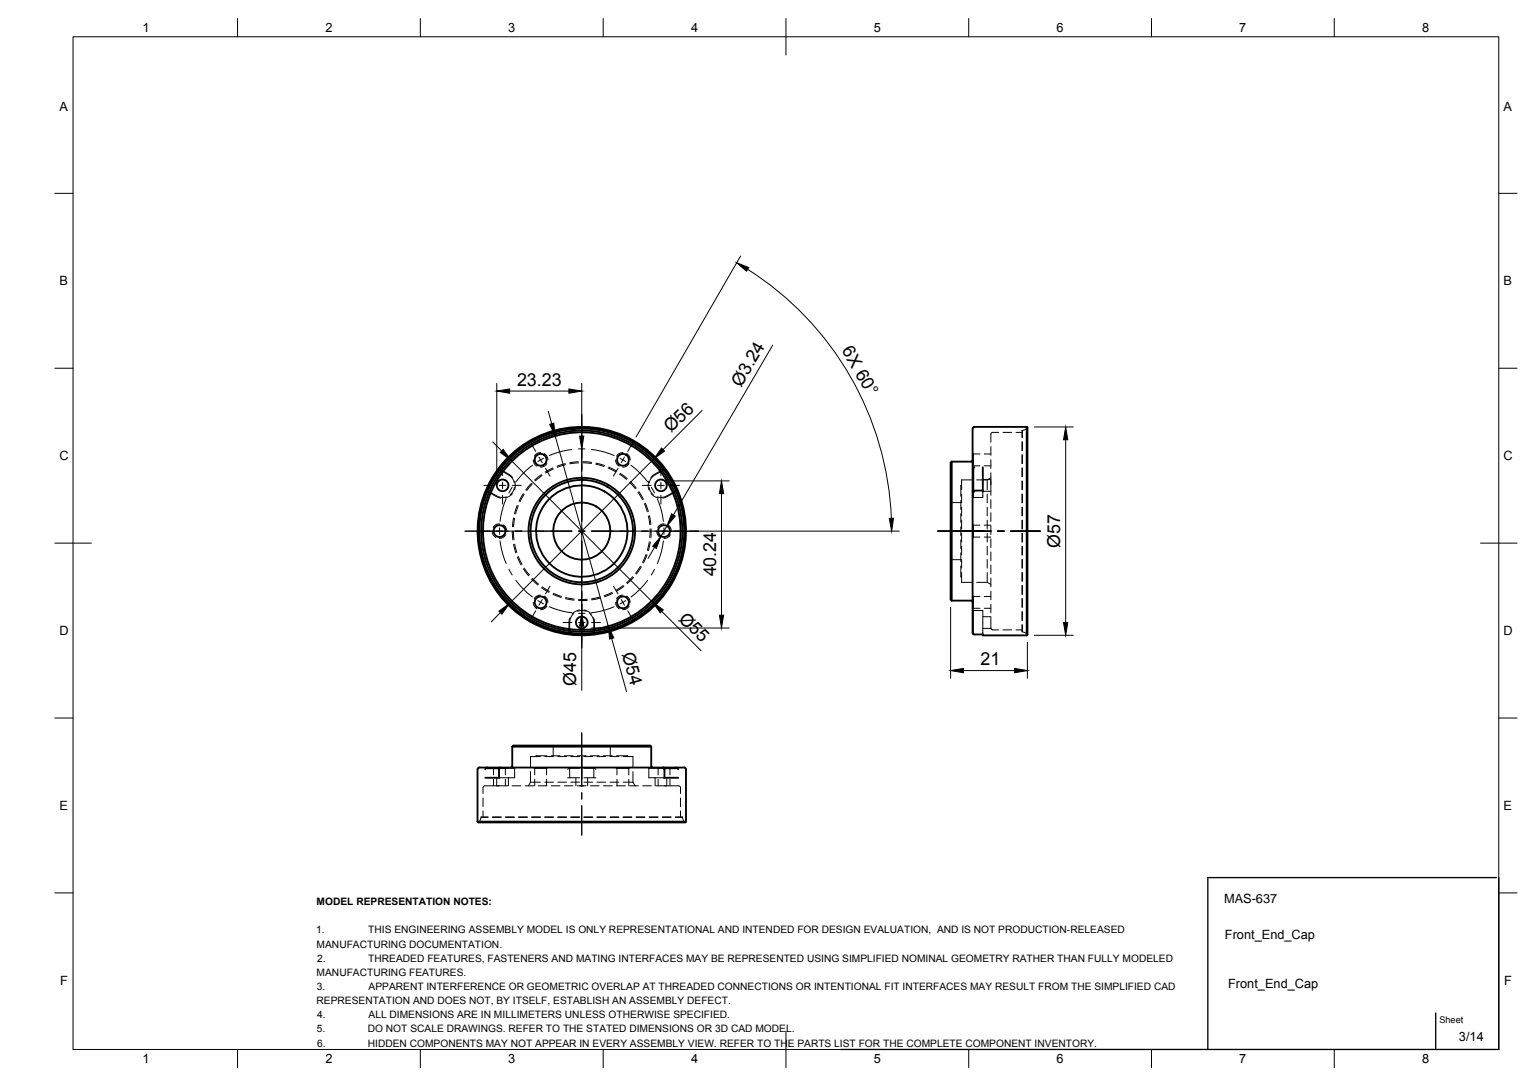
ISO-10303-21;
HEADER;
FILE_DESCRIPTION((''),'2;1');
FILE_NAME('Front_End_Cap.step','2026-10-09T10:11:57-07:00',(''),(''),'','','');
FILE_SCHEMA (('AUTOMOTIVE_DESIGN { 1 0 10303 214 3 1 1 }'));
ENDSEC;
DATA;
#10=MECHANICAL_DESIGN_GEOMETRIC_PRESENTATION_REPRESENTATION('',(#123),#13510);
#93=SHAPE_REPRESENTATION_RELATIONSHIP('SRR','None',#13563,#108) ;
#108=ADVANCED_BREP_SHAPE_REPRESENTATION('',(#155),#13495) ;
#123=STYLED_ITEM('',(#13647),#155) ;
#155=MANIFOLD_SOLID_BREP('Body1',#7372) ;
#187=ELLIPSE('',#7677,0.707106781186342,0.5) ;
#188=ELLIPSE('',#7688,0.707106781186342,0.5) ;
#189=ELLIPSE('',#7692,0.707106781186342,0.5) ;
#190=ELLIPSE('',#7702,0.707106781186342,0.5) ;
#191=ELLIPSE('',#7709,0.707106781186548,0.5) ;
#192=ELLIPSE('',#7716,0.707106781186548,0.5) ;
#193=FACE_BOUND('',#1127,.T.) ;
#194=FACE_BOUND('',#1131,.T.) ;
#195=FACE_BOUND('',#1137,.T.) ;
#196=FACE_BOUND('',#1140,.T.) ;
#197=FACE_BOUND('',#1143,.T.) ;
#198=FACE_BOUND('',#1150,.T.) ;
#199=FACE_BOUND('',#1151,.T.) ;
#200=FACE_BOUND('',#1152,.T.) ;
#201=FACE_BOUND('',#1153,.T.) ;
#202=FACE_BOUND('',#1154,.T.) ;
#203=FACE_BOUND('',#1155,.T.) ;
#204=FACE_BOUND('',#1156,.T.) ;
#205=FACE_BOUND('',#1173,.T.) ;
#206=FACE_BOUND('',#1174,.T.) ;
#207=FACE_BOUND('',#1175,.T.) ;
#208=FACE_BOUND('',#1176,.T.) ;
#209=FACE_BOUND('',#1177,.T.) ;
#210=FACE_BOUND('',#1178,.T.) ;
#211=FACE_BOUND('',#1179,.T.) ;
#212=FACE_BOUND('',#1185,.T.) ;
#213=FACE_BOUND('',#1194,.T.) ;
#214=FACE_BOUND('',#1204,.T.) ;
#266=PLANE('',#7586) ;
#267=PLANE('',#7592) ;
#268=PLANE('',#7604) ;
#269=PLANE('',#7608) ;
#270=PLANE('',#7612) ;
#271=PLANE('',#7630) ;
#272=PLANE('',#7669) ;
#273=PLANE('',#7675) ;
#274=PLANE('',#7676) ;
#275=PLANE('',#7680) ;
#276=PLANE('',#7686) ;
#277=PLANE('',#7687) ;
#278=PLANE('',#7690) ;
#279=PLANE('',#7691) ;
#280=PLANE('',#7695) ;
#281=PLANE('',#7700) ;
#282=PLANE('',#7701) ;
#283=PLANE('',#7707) ;
#284=PLANE('',#7708) ;
#285=PLANE('',#7712) ;
#286=PLANE('',#7714) ;
#287=PLANE('',#7715) ;
#474=B_SPLINE_CURVE_WITH_KNOTS('',3,(#11072,#11073,#11074,#11075,#11076,
#11077,#11078,#11079,#11080,#11081,#11082,#11083,#11084,#11085,#11086,#11087,
#11088,#11089,#11090,#11091,#11092,#11093),.UNSPECIFIED.,.F.,.F.,(4,2,2,
2,2,2,2,2,2,2,4),(-0.52146341780892,-0.494765818804412,-0.469284384601152,
-0.465421081717763,-0.463705360184221,-0.462435620950771,-0.461259293496834,
-0.45965735667046,-0.455678085608089,-0.412270185488608,-0.400473329912757),
 .UNSPECIFIED.) ;
#475=B_SPLINE_CURVE_WITH_KNOTS('',3,(#11097,#11098,#11099,#11100,#11101,
#11102,#11103,#11104,#11105,#11106,#11107,#11108,#11109,#11110,#11111,#11112,
#11113,#11114,#11115,#11116,#11117,#11118),.UNSPECIFIED.,.F.,.F.,(4,2,2,
2,2,2,2,2,2,2,4),(-0.521463417334395,-0.49476581835854,-0.469284384179659,
-0.465421081300331,-0.463705359768128,-0.462435620535193,-0.461259293081839,
-0.459657356256884,-0.455678085198087,-0.412270185114522,-0.400473329554445),
 .UNSPECIFIED.) ;
#476=B_SPLINE_CURVE_WITH_KNOTS('',3,(#11122,#11123,#11124,#11125,#11126,
#11127,#11128,#11129,#11130,#11131,#11132,#11133,#11134,#11135,#11136,#11137,
#11138,#11139,#11140,#11141,#11142,#11143),.UNSPECIFIED.,.F.,.F.,(4,2,2,
2,2,2,2,2,2,2,4),(-0.521463417713865,-0.494765818712896,-0.469284384508709,
-0.46542108162507,-0.463705360091333,-0.462435620857346,-0.461259293403164,
-0.459657356577429,-0.455678085515946,-0.412270185406787,-0.400473329829023),
 .UNSPECIFIED.) ;
#477=B_SPLINE_CURVE_WITH_KNOTS('',3,(#11350,#11351,#11352,#11353,#11354,
#11355),.UNSPECIFIED.,.F.,.F.,(4,2,4),(0.26873156819099,0.285572320159818,
0.298230301897838),.UNSPECIFIED.) ;
#478=B_SPLINE_CURVE_WITH_KNOTS('',3,(#11361,#11362,#11363,#11364,#11365,
#11366,#11367,#11368,#11369,#11370,#11371,#11372),.UNSPECIFIED.,.F.,.F.,
(4,2,2,2,2,4),(-0.000449132348290775,2.53732061403222E-12,0.0221149603912549,
0.0431990642467605,0.06500366116372,0.0651070090170544),.UNSPECIFIED.) ;
#479=B_SPLINE_CURVE_WITH_KNOTS('',3,(#11385,#11386,#11387,#11388,#11389,
#11390,#11391,#11392,#11393,#11394,#11395,#11396),.UNSPECIFIED.,.F.,.F.,
(4,2,2,2,2,4),(-0.000449133003127626,1.85615813084322E-12,0.0221149611703719,
0.0431990661916226,0.065003665298961,0.0651070140798856),.UNSPECIFIED.) ;
#480=B_SPLINE_CURVE_WITH_KNOTS('',3,(#11397,#11398,#11399,#11400,#11401,
#11402),.UNSPECIFIED.,.F.,.F.,(4,2,4),(-0.0927109544955969,-0.0758702025273432,
-0.0632122207848772),.UNSPECIFIED.) ;
#481=B_SPLINE_CURVE_WITH_KNOTS('',3,(#11404,#11405,#11406,#11407,#11408,
#11409),.UNSPECIFIED.,.F.,.F.,(4,2,4),(0.268765463242126,0.285606215210891,
0.298264196947108),.UNSPECIFIED.) ;
#482=B_SPLINE_CURVE_WITH_KNOTS('',3,(#11411,#11412,#11413,#11414,#11415,
#11416,#11417,#11418,#11419,#11420,#11421,#11422),.UNSPECIFIED.,.F.,.F.,
(4,2,2,2,2,4),(-0.22538340226828,-0.224833171566157,-0.19774023813781,-0.171910201657709,
-0.145197491309789,-0.145070879202733),.UNSPECIFIED.) ;
#483=B_SPLINE_CURVE_WITH_KNOTS('',3,(#11455,#11456,#11457,#11458,#11459,
#11460,#11461,#11462,#11463,#11464,#11465,#11466),.UNSPECIFIED.,.F.,.F.,
(4,2,2,2,2,4),(-0.000449132829525576,1.42051192857096E-13,0.0221149610887194,
0.0431990659374438,0.0650036645796739,0.0651070130619044),.UNSPECIFIED.) ;
#484=B_SPLINE_CURVE_WITH_KNOTS('',3,(#11467,#11468,#11469,#11470,#11471,
#11472),.UNSPECIFIED.,.F.,.F.,(4,2,4),(-0.0927109544901547,-0.0758702025249889,
-0.0632122207639069),.UNSPECIFIED.) ;
#485=B_SPLINE_CURVE_WITH_KNOTS('',3,(#11474,#11475,#11476,#11477,#11478,
#11479),.UNSPECIFIED.,.F.,.F.,(4,2,4),(0.268731568191897,0.285572320160214,
0.298230301904486),.UNSPECIFIED.) ;
#486=B_SPLINE_CURVE_WITH_KNOTS('',3,(#11480,#11481,#11482,#11483,#11484,
#11485,#11486,#11487,#11488,#11489,#11490,#11491),.UNSPECIFIED.,.F.,.F.,
(4,2,2,2,2,4),(-0.225383330725163,-0.224833100967517,-0.197740175527576,
-0.171910147180953,-0.145197446451029,-0.145070835530411),.UNSPECIFIED.) ;
#487=B_SPLINE_CURVE_WITH_KNOTS('',3,(#11529,#11530,#11531,#11532,#11533,
#11534),.UNSPECIFIED.,.F.,.F.,(4,2,4),(-0.0927254732348807,-0.0743662922611468,
-0.0631177306127901),.UNSPECIFIED.) ;
#488=B_SPLINE_CURVE_WITH_KNOTS('',3,(#11537,#11538,#11539,#11540,#11541,
#11542,#11543,#11544,#11545,#11546,#11547,#11548),.UNSPECIFIED.,.F.,.F.,
(4,2,2,2,2,4),(-0.225383401816229,-0.224833171320864,-0.197740237586304,
-0.171910200932329,-0.145197490755643,-0.145070879020991),.UNSPECIFIED.) ;
#492=TOROIDAL_SURFACE('',#7577,26.5,0.5) ;
#493=TOROIDAL_SURFACE('',#7596,19.4,0.4) ;
#494=TOROIDAL_SURFACE('',#7683,28.,0.5) ;
#495=TOROIDAL_SURFACE('',#7698,28.,0.5) ;
#496=TOROIDAL_SURFACE('',#7717,28.,0.5) ;
#541=CYLINDRICAL_SURFACE('',#7575,1.621) ;
#542=CYLINDRICAL_SURFACE('',#7584,27.) ;
#543=CYLINDRICAL_SURFACE('',#7588,27.5) ;
#544=CYLINDRICAL_SURFACE('',#7600,19.) ;
#545=CYLINDRICAL_SURFACE('',#7606,7.8) ;
#546=CYLINDRICAL_SURFACE('',#7610,12.5) ;
#547=CYLINDRICAL_SURFACE('',#7614,14.) ;
#548=CYLINDRICAL_SURFACE('',#7618,1.6) ;
#549=CYLINDRICAL_SURFACE('',#7622,1.6) ;
#550=CYLINDRICAL_SURFACE('',#7626,1.6) ;
#551=CYLINDRICAL_SURFACE('',#7639,1.621) ;
#552=CYLINDRICAL_SURFACE('',#7643,1.621) ;
#553=CYLINDRICAL_SURFACE('',#7647,1.621) ;
#554=CYLINDRICAL_SURFACE('',#7651,1.621) ;
#555=CYLINDRICAL_SURFACE('',#7655,1.621) ;
#556=CYLINDRICAL_SURFACE('',#7656,3.3) ;
#557=CYLINDRICAL_SURFACE('',#7661,3.3) ;
#558=CYLINDRICAL_SURFACE('',#7666,3.3) ;
#559=CYLINDRICAL_SURFACE('',#7678,0.5) ;
#560=CYLINDRICAL_SURFACE('',#7689,0.5) ;
#561=CYLINDRICAL_SURFACE('',#7693,0.5) ;
#562=CYLINDRICAL_SURFACE('',#7703,28.5) ;
#563=CYLINDRICAL_SURFACE('',#7706,0.5) ;
#564=CYLINDRICAL_SURFACE('',#7710,0.5) ;
#565=CYLINDRICAL_SURFACE('',#7718,0.5) ;
#668=FACE_OUTER_BOUND('',#1122,.T.) ;
#669=FACE_OUTER_BOUND('',#1123,.T.) ;
#670=FACE_OUTER_BOUND('',#1124,.T.) ;
#671=FACE_OUTER_BOUND('',#1125,.T.) ;
#672=FACE_OUTER_BOUND('',#1126,.T.) ;
#673=FACE_OUTER_BOUND('',#1128,.T.) ;
#674=FACE_OUTER_BOUND('',#1129,.T.) ;
#675=FACE_OUTER_BOUND('',#1130,.T.) ;
#676=FACE_OUTER_BOUND('',#1132,.T.) ;
#677=FACE_OUTER_BOUND('',#1133,.T.) ;
#678=FACE_OUTER_BOUND('',#1134,.T.) ;
#679=FACE_OUTER_BOUND('',#1135,.T.) ;
#680=FACE_OUTER_BOUND('',#1136,.T.) ;
#681=FACE_OUTER_BOUND('',#1138,.T.) ;
#682=FACE_OUTER_BOUND('',#1139,.T.) ;
#683=FACE_OUTER_BOUND('',#1141,.T.) ;
#684=FACE_OUTER_BOUND('',#1142,.T.) ;
#685=FACE_OUTER_BOUND('',#1144,.T.) ;
#686=FACE_OUTER_BOUND('',#1145,.T.) ;
#687=FACE_OUTER_BOUND('',#1146,.T.) ;
#688=FACE_OUTER_BOUND('',#1147,.T.) ;
#689=FACE_OUTER_BOUND('',#1148,.T.) ;
#690=FACE_OUTER_BOUND('',#1149,.T.) ;
#691=FACE_OUTER_BOUND('',#1157,.T.) ;
#692=FACE_OUTER_BOUND('',#1158,.T.) ;
#693=FACE_OUTER_BOUND('',#1159,.T.) ;
#694=FACE_OUTER_BOUND('',#1160,.T.) ;
#695=FACE_OUTER_BOUND('',#1161,.T.) ;
#696=FACE_OUTER_BOUND('',#1162,.T.) ;
#697=FACE_OUTER_BOUND('',#1163,.T.) ;
#698=FACE_OUTER_BOUND('',#1164,.T.) ;
#699=FACE_OUTER_BOUND('',#1165,.T.) ;
#700=FACE_OUTER_BOUND('',#1166,.T.) ;
#701=FACE_OUTER_BOUND('',#1167,.T.) ;
#702=FACE_OUTER_BOUND('',#1168,.T.) ;
#703=FACE_OUTER_BOUND('',#1169,.T.) ;
#704=FACE_OUTER_BOUND('',#1170,.T.) ;
#705=FACE_OUTER_BOUND('',#1171,.T.) ;
#706=FACE_OUTER_BOUND('',#1172,.T.) ;
#707=FACE_OUTER_BOUND('',#1180,.T.) ;
#708=FACE_OUTER_BOUND('',#1181,.T.) ;
#709=FACE_OUTER_BOUND('',#1182,.T.) ;
#710=FACE_OUTER_BOUND('',#1183,.T.) ;
#711=FACE_OUTER_BOUND('',#1184,.T.) ;
#712=FACE_OUTER_BOUND('',#1186,.T.) ;
#713=FACE_OUTER_BOUND('',#1187,.T.) ;
#714=FACE_OUTER_BOUND('',#1188,.T.) ;
#715=FACE_OUTER_BOUND('',#1189,.T.) ;
#716=FACE_OUTER_BOUND('',#1190,.T.) ;
#717=FACE_OUTER_BOUND('',#1191,.T.) ;
#718=FACE_OUTER_BOUND('',#1192,.T.) ;
#719=FACE_OUTER_BOUND('',#1193,.T.) ;
#720=FACE_OUTER_BOUND('',#1195,.T.) ;
#721=FACE_OUTER_BOUND('',#1196,.T.) ;
#722=FACE_OUTER_BOUND('',#1197,.T.) ;
#723=FACE_OUTER_BOUND('',#1198,.T.) ;
#724=FACE_OUTER_BOUND('',#1199,.T.) ;
#725=FACE_OUTER_BOUND('',#1200,.T.) ;
#726=FACE_OUTER_BOUND('',#1201,.T.) ;
#727=FACE_OUTER_BOUND('',#1202,.T.) ;
#728=FACE_OUTER_BOUND('',#1203,.T.) ;
#729=FACE_OUTER_BOUND('',#1205,.T.) ;
#730=FACE_OUTER_BOUND('',#1206,.T.) ;
#731=FACE_OUTER_BOUND('',#1207,.T.) ;
#732=FACE_OUTER_BOUND('',#1208,.T.) ;
#1122=EDGE_LOOP('',(#4822,#4823,#4824,#4825)) ;
#1123=EDGE_LOOP('',(#4826,#4827,#4828,#4829)) ;
#1124=EDGE_LOOP('',(#4830,#4831,#4832,#4833,#4834,#4835,#4836,#4837,#4838,
#4839)) ;
#1125=EDGE_LOOP('',(#4840,#4841,#4842,#4843)) ;
#1126=EDGE_LOOP('',(#4844)) ;
#1127=EDGE_LOOP('',(#4845)) ;
#1128=EDGE_LOOP('',(#4846,#4847,#4848,#4849)) ;
#1129=EDGE_LOOP('',(#4850,#4851,#4852,#4853)) ;
#1130=EDGE_LOOP('',(#4854)) ;
#1131=EDGE_LOOP('',(#4855)) ;
#1132=EDGE_LOOP('',(#4856,#4857,#4858,#4859)) ;
#1133=EDGE_LOOP('',(#4860,#4861,#4862,#4863)) ;
#1134=EDGE_LOOP('',(#4864,#4865,#4866,#4867)) ;
#1135=EDGE_LOOP('',(#4868,#4869,#4870,#4871)) ;
#1136=EDGE_LOOP('',(#4872)) ;
#1137=EDGE_LOOP('',(#4873)) ;
#1138=EDGE_LOOP('',(#4874,#4875,#4876,#4877)) ;
#1139=EDGE_LOOP('',(#4878)) ;
#1140=EDGE_LOOP('',(#4879)) ;
#1141=EDGE_LOOP('',(#4880,#4881,#4882,#4883)) ;
#1142=EDGE_LOOP('',(#4884)) ;
#1143=EDGE_LOOP('',(#4885)) ;
#1144=EDGE_LOOP('',(#4886,#4887,#4888,#4889)) ;
#1145=EDGE_LOOP('',(#4890,#4891,#4892,#4893)) ;
#1146=EDGE_LOOP('',(#4894,#4895,#4896,#4897,#4898,#4899)) ;
#1147=EDGE_LOOP('',(#4900,#4901,#4902,#4903,#4904,#4905)) ;
#1148=EDGE_LOOP('',(#4906,#4907,#4908,#4909,#4910,#4911)) ;
#1149=EDGE_LOOP('',(#4912,#4913,#4914,#4915,#4916,#4917,#4918,#4919,#4920,
#4921)) ;
#1150=EDGE_LOOP('',(#4922)) ;
#1151=EDGE_LOOP('',(#4923)) ;
#1152=EDGE_LOOP('',(#4924)) ;
#1153=EDGE_LOOP('',(#4925)) ;
#1154=EDGE_LOOP('',(#4926)) ;
#1155=EDGE_LOOP('',(#4927)) ;
#1156=EDGE_LOOP('',(#4928)) ;
#1157=EDGE_LOOP('',(#4929,#4930,#4931,#4932)) ;
#1158=EDGE_LOOP('',(#4933,#4934,#4935,#4936)) ;
#1159=EDGE_LOOP('',(#4937,#4938,#4939,#4940)) ;
#1160=EDGE_LOOP('',(#4941,#4942,#4943,#4944)) ;
#1161=EDGE_LOOP('',(#4945,#4946,#4947,#4948)) ;
#1162=EDGE_LOOP('',(#4949,#4950,#4951,#4952)) ;
#1163=EDGE_LOOP('',(#4953,#4954,#4955,#4956)) ;
#1164=EDGE_LOOP('',(#4957,#4958,#4959,#4960)) ;
#1165=EDGE_LOOP('',(#4961,#4962,#4963,#4964)) ;
#1166=EDGE_LOOP('',(#4965,#4966,#4967,#4968)) ;
#1167=EDGE_LOOP('',(#4969,#4970,#4971,#4972)) ;
#1168=EDGE_LOOP('',(#4973,#4974,#4975,#4976)) ;
#1169=EDGE_LOOP('',(#4977,#4978,#4979,#4980)) ;
#1170=EDGE_LOOP('',(#4981,#4982,#4983,#4984)) ;
#1171=EDGE_LOOP('',(#4985,#4986,#4987,#4988)) ;
#1172=EDGE_LOOP('',(#4989,#4990,#4991,#4992,#4993,#4994,#4995,#4996,#4997,
#4998,#4999,#5000)) ;
#1173=EDGE_LOOP('',(#5001)) ;
#1174=EDGE_LOOP('',(#5002)) ;
#1175=EDGE_LOOP('',(#5003)) ;
#1176=EDGE_LOOP('',(#5004)) ;
#1177=EDGE_LOOP('',(#5005)) ;
#1178=EDGE_LOOP('',(#5006)) ;
#1179=EDGE_LOOP('',(#5007)) ;
#1180=EDGE_LOOP('',(#5008,#5009,#5010,#5011)) ;
#1181=EDGE_LOOP('',(#5012,#5013,#5014,#5015)) ;
#1182=EDGE_LOOP('',(#5016,#5017,#5018,#5019,#5020)) ;
#1183=EDGE_LOOP('',(#5021,#5022,#5023,#5024,#5025)) ;
#1184=EDGE_LOOP('',(#5026,#5027,#5028,#5029,#5030,#5031)) ;
#1185=EDGE_LOOP('',(#5032)) ;
#1186=EDGE_LOOP('',(#5033,#5034,#5035,#5036,#5037,#5038,#5039)) ;
#1187=EDGE_LOOP('',(#5040,#5041,#5042,#5043)) ;
#1188=EDGE_LOOP('',(#5044,#5045,#5046,#5047,#5048)) ;
#1189=EDGE_LOOP('',(#5049,#5050,#5051,#5052,#5053)) ;
#1190=EDGE_LOOP('',(#5054,#5055,#5056,#5057)) ;
#1191=EDGE_LOOP('',(#5058,#5059,#5060,#5061,#5062)) ;
#1192=EDGE_LOOP('',(#5063,#5064,#5065,#5066,#5067)) ;
#1193=EDGE_LOOP('',(#5068,#5069,#5070,#5071,#5072,#5073)) ;
#1194=EDGE_LOOP('',(#5074)) ;
#1195=EDGE_LOOP('',(#5075,#5076,#5077,#5078,#5079,#5080)) ;
#1196=EDGE_LOOP('',(#5081,#5082,#5083,#5084)) ;
#1197=EDGE_LOOP('',(#5085,#5086,#5087,#5088,#5089)) ;
#1198=EDGE_LOOP('',(#5090,#5091,#5092,#5093,#5094,#5095,#5096,#5097,#5098,
#5099,#5100,#5101,#5102,#5103,#5104,#5105)) ;
#1199=EDGE_LOOP('',(#5106,#5107,#5108,#5109,#5110)) ;
#1200=EDGE_LOOP('',(#5111,#5112,#5113,#5114)) ;
#1201=EDGE_LOOP('',(#5115,#5116,#5117,#5118,#5119)) ;
#1202=EDGE_LOOP('',(#5120,#5121,#5122,#5123,#5124)) ;
#1203=EDGE_LOOP('',(#5125,#5126,#5127,#5128,#5129,#5130)) ;
#1204=EDGE_LOOP('',(#5131)) ;
#1205=EDGE_LOOP('',(#5132,#5133,#5134,#5135)) ;
#1206=EDGE_LOOP('',(#5136,#5137,#5138,#5139,#5140)) ;
#1207=EDGE_LOOP('',(#5141,#5142,#5143,#5144,#5145,#5146)) ;
#1208=EDGE_LOOP('',(#5147,#5148,#5149,#5150,#5151)) ;
#1649=LINE('',#11061,#2143) ;
#1650=LINE('',#11065,#2144) ;
#1651=LINE('',#11150,#2145) ;
#1652=LINE('',#11157,#2146) ;
#1653=LINE('',#11161,#2147) ;
#1654=LINE('',#11169,#2148) ;
#1655=LINE('',#11178,#2149) ;
#1656=LINE('',#11182,#2150) ;
#1657=LINE('',#11189,#2151) ;
#1658=LINE('',#11196,#2152) ;
#1659=LINE('',#11203,#2153) ;
#1660=LINE('',#11207,#2154) ;
#1661=LINE('',#11213,#2155) ;
#1662=LINE('',#11220,#2156) ;
#1663=LINE('',#11227,#2157) ;
#1664=LINE('',#11245,#2158) ;
#1665=LINE('',#11248,#2159) ;
#1666=LINE('',#11253,#2160) ;
#1667=LINE('',#11256,#2161) ;
#1668=LINE('',#11261,#2162) ;
#1669=LINE('',#11264,#2163) ;
#1670=LINE('',#11269,#2164) ;
#1671=LINE('',#11272,#2165) ;
#1672=LINE('',#11277,#2166) ;
#1673=LINE('',#11280,#2167) ;
#1674=LINE('',#11286,#2168) ;
#1675=LINE('',#11289,#2169) ;
#1676=LINE('',#11292,#2170) ;
#1677=LINE('',#11294,#2171) ;
#1678=LINE('',#11301,#2172) ;
#1679=LINE('',#11304,#2173) ;
#1680=LINE('',#11307,#2174) ;
#1681=LINE('',#11309,#2175) ;
#1682=LINE('',#11316,#2176) ;
#1683=LINE('',#11319,#2177) ;
#1684=LINE('',#11323,#2178) ;
#1685=LINE('',#11327,#2179) ;
#1686=LINE('',#11330,#2180) ;
#1687=LINE('',#11332,#2181) ;
#1688=LINE('',#11335,#2182) ;
#1689=LINE('',#11337,#2183) ;
#1690=LINE('',#11340,#2184) ;
#1691=LINE('',#11341,#2185) ;
#1692=LINE('',#11344,#2186) ;
#1693=LINE('',#11346,#2187) ;
#1694=LINE('',#11347,#2188) ;
#1695=LINE('',#11373,#2189) ;
#1696=LINE('',#11376,#2190) ;
#1697=LINE('',#11426,#2191) ;
#1698=LINE('',#11427,#2192) ;
#1699=LINE('',#11431,#2193) ;
#1700=LINE('',#11434,#2194) ;
#1701=LINE('',#11436,#2195) ;
#1702=LINE('',#11437,#2196) ;
#1703=LINE('',#11443,#2197) ;
#1704=LINE('',#11446,#2198) ;
#1705=LINE('',#11494,#2199) ;
#1706=LINE('',#11495,#2200) ;
#1707=LINE('',#11499,#2201) ;
#1708=LINE('',#11503,#2202) ;
#1709=LINE('',#11506,#2203) ;
#1710=LINE('',#11507,#2204) ;
#1711=LINE('',#11511,#2205) ;
#1712=LINE('',#11513,#2206) ;
#1713=LINE('',#11514,#2207) ;
#1714=LINE('',#11521,#2208) ;
#1715=LINE('',#11525,#2209) ;
#1716=LINE('',#11526,#2210) ;
#2143=VECTOR('',#8575,1.621) ;
#2144=VECTOR('',#8580,1.621) ;
#2145=VECTOR('',#8599,27.) ;
#2146=VECTOR('',#8608,27.5) ;
#2147=VECTOR('',#8613,27.5) ;
#2148=VECTOR('',#8624,28.3) ;
#2149=VECTOR('',#8635,19.) ;
#2150=VECTOR('',#8640,18.7) ;
#2151=VECTOR('',#8649,7.8) ;
#2152=VECTOR('',#8658,12.5) ;
#2153=VECTOR('',#8667,14.) ;
#2154=VECTOR('',#8672,14.) ;
#2155=VECTOR('',#8679,1.6) ;
#2156=VECTOR('',#8688,1.6) ;
#2157=VECTOR('',#8697,1.6) ;
#2158=VECTOR('',#8718,1.621) ;
#2159=VECTOR('',#8723,1.621) ;
#2160=VECTOR('',#8728,1.621) ;
#2161=VECTOR('',#8733,1.621) ;
#2162=VECTOR('',#8738,1.621) ;
#2163=VECTOR('',#8743,1.621) ;
#2164=VECTOR('',#8748,1.621) ;
#2165=VECTOR('',#8753,1.621) ;
#2166=VECTOR('',#8758,1.621) ;
#2167=VECTOR('',#8763,1.621) ;
#2168=VECTOR('',#8768,1.) ;
#2169=VECTOR('',#8771,1.) ;
#2170=VECTOR('',#8774,0.999999999999642) ;
#2171=VECTOR('',#8775,1.00000000000035) ;
#2172=VECTOR('',#8782,1.) ;
#2173=VECTOR('',#8785,1.) ;
#2174=VECTOR('',#8788,0.999999999999642) ;
#2175=VECTOR('',#8789,0.999999999999901) ;
#2176=VECTOR('',#8796,1.) ;
#2177=VECTOR('',#8799,1.) ;
#2178=VECTOR('',#8802,1.) ;
#2179=VECTOR('',#8805,1.) ;
#2180=VECTOR('',#8808,0.99999999999962) ;
#2181=VECTOR('',#8809,0.99999999999962) ;
#2182=VECTOR('',#8812,0.99999999999962) ;
#2183=VECTOR('',#8813,0.99999999999962) ;
#2184=VECTOR('',#8818,0.999999999999933) ;
#2185=VECTOR('',#8819,0.999999999999933) ;
#2186=VECTOR('',#8822,0.99999999999962) ;
#2187=VECTOR('',#8823,0.99999999999962) ;
#2188=VECTOR('',#8824,1.) ;
#2189=VECTOR('',#8833,1.) ;
#2190=VECTOR('',#8836,0.99999999999962) ;
#2191=VECTOR('',#8849,0.99999999999962) ;
#2192=VECTOR('',#8850,1.) ;
#2193=VECTOR('',#8857,1.) ;
#2194=VECTOR('',#8860,0.99999999999962) ;
#2195=VECTOR('',#8861,0.99999999999962) ;
#2196=VECTOR('',#8862,1.) ;
#2197=VECTOR('',#8871,1.) ;
#2198=VECTOR('',#8874,0.99999999999962) ;
#2199=VECTOR('',#8885,0.99999999999962) ;
#2200=VECTOR('',#8886,1.) ;
#2201=VECTOR('',#8893,28.5) ;
#2202=VECTOR('',#8896,1.) ;
#2203=VECTOR('',#8899,1.) ;
#2204=VECTOR('',#8900,1.) ;
#2205=VECTOR('',#8905,1.) ;
#2206=VECTOR('',#8906,1.) ;
#2207=VECTOR('',#8907,1.) ;
#2208=VECTOR('',#8918,1.) ;
#2209=VECTOR('',#8923,1.) ;
#2210=VECTOR('',#8924,1.) ;
#2637=CIRCLE('',#7573,1.621) ;
#2638=CIRCLE('',#7574,2.) ;
#2639=CIRCLE('',#7576,1.621) ;
#2640=CIRCLE('',#7578,26.5) ;
#2641=CIRCLE('',#7579,26.5) ;
#2642=CIRCLE('',#7580,26.5) ;
#2643=CIRCLE('',#7581,26.5) ;
#2644=CIRCLE('',#7582,0.5) ;
#2645=CIRCLE('',#7583,27.) ;
#2646=CIRCLE('',#7585,27.) ;
#2647=CIRCLE('',#7587,27.5) ;
#2648=CIRCLE('',#7589,27.5) ;
#2649=CIRCLE('',#7591,28.) ;
#2650=CIRCLE('',#7593,28.3) ;
#2651=CIRCLE('',#7595,28.5) ;
#2652=CIRCLE('',#7597,19.4) ;
#2653=CIRCLE('',#7598,0.4) ;
#2654=CIRCLE('',#7599,19.) ;
#2655=CIRCLE('',#7601,19.) ;
#2656=CIRCLE('',#7603,18.7) ;
#2657=CIRCLE('',#7605,7.8) ;
#2658=CIRCLE('',#7607,7.8) ;
#2659=CIRCLE('',#7609,12.5) ;
#2660=CIRCLE('',#7611,12.5) ;
#2661=CIRCLE('',#7613,14.) ;
#2662=CIRCLE('',#7615,14.) ;
#2663=CIRCLE('',#7617,14.5773502692) ;
#2664=CIRCLE('',#7619,1.6) ;
#2665=CIRCLE('',#7620,1.6) ;
#2666=CIRCLE('',#7621,1.6) ;
#2667=CIRCLE('',#7623,1.6) ;
#2668=CIRCLE('',#7624,1.6) ;
#2669=CIRCLE('',#7625,1.6) ;
#2670=CIRCLE('',#7627,1.6) ;
#2671=CIRCLE('',#7628,1.6) ;
#2672=CIRCLE('',#7629,1.6) ;
#2673=CIRCLE('',#7631,1.621) ;
#2674=CIRCLE('',#7632,1.621) ;
#2675=CIRCLE('',#7633,1.621) ;
#2676=CIRCLE('',#7634,1.621) ;
#2677=CIRCLE('',#7635,1.621) ;
#2678=CIRCLE('',#7637,1.621) ;
#2679=CIRCLE('',#7638,2.) ;
#2680=CIRCLE('',#7641,1.621) ;
#2681=CIRCLE('',#7642,2.) ;
#2682=CIRCLE('',#7645,1.621) ;
#2683=CIRCLE('',#7646,2.) ;
#2684=CIRCLE('',#7649,1.621) ;
#2685=CIRCLE('',#7650,2.) ;
#2686=CIRCLE('',#7653,1.621) ;
#2687=CIRCLE('',#7654,2.) ;
#2688=CIRCLE('',#7657,3.3) ;
#2689=CIRCLE('',#7658,3.3) ;
#2690=CIRCLE('',#7660,3.5) ;
#2691=CIRCLE('',#7662,3.3) ;
#2692=CIRCLE('',#7663,3.3) ;
#2693=CIRCLE('',#7665,3.5) ;
#2694=CIRCLE('',#7667,3.3) ;
#2695=CIRCLE('',#7668,3.3) ;
#2696=CIRCLE('',#7670,3.5) ;
#2697=CIRCLE('',#7671,28.) ;
#2698=CIRCLE('',#7672,28.) ;
#2699=CIRCLE('',#7673,28.) ;
#2700=CIRCLE('',#7679,0.5) ;
#2701=CIRCLE('',#7681,28.5) ;
#2702=CIRCLE('',#7682,0.5) ;
#2703=CIRCLE('',#7684,28.5) ;
#2704=CIRCLE('',#7685,28.5) ;
#2705=CIRCLE('',#7694,0.5) ;
#2706=CIRCLE('',#7696,28.5) ;
#2707=CIRCLE('',#7697,0.5) ;
#2708=CIRCLE('',#7699,28.5) ;
#2709=CIRCLE('',#7704,28.5) ;
#2710=CIRCLE('',#7705,28.5) ;
#2711=CIRCLE('',#7711,0.5) ;
#2712=CIRCLE('',#7713,0.5) ;
#3143=VERTEX_POINT('',#11058) ;
#3144=VERTEX_POINT('',#11060) ;
#3145=VERTEX_POINT('',#11064) ;
#3146=VERTEX_POINT('',#11068) ;
#3147=VERTEX_POINT('',#11069) ;
#3148=VERTEX_POINT('',#11071) ;
#3149=VERTEX_POINT('',#11094) ;
#3150=VERTEX_POINT('',#11096) ;
#3151=VERTEX_POINT('',#11119) ;
#3152=VERTEX_POINT('',#11121) ;
#3153=VERTEX_POINT('',#11145) ;
#3154=VERTEX_POINT('',#11149) ;
#3155=VERTEX_POINT('',#11153) ;
#3156=VERTEX_POINT('',#11156) ;
#3157=VERTEX_POINT('',#11160) ;
#3158=VERTEX_POINT('',#11164) ;
#3159=VERTEX_POINT('',#11167) ;
#3160=VERTEX_POINT('',#11171) ;
#3161=VERTEX_POINT('',#11173) ;
#3162=VERTEX_POINT('',#11177) ;
#3163=VERTEX_POINT('',#11181) ;
#3164=VERTEX_POINT('',#11185) ;
#3165=VERTEX_POINT('',#11188) ;
#3166=VERTEX_POINT('',#11192) ;
#3167=VERTEX_POINT('',#11195) ;
#3168=VERTEX_POINT('',#11199) ;
#3169=VERTEX_POINT('',#11202) ;
#3170=VERTEX_POINT('',#11206) ;
#3171=VERTEX_POINT('',#11210) ;
#3172=VERTEX_POINT('',#11212) ;
#3173=VERTEX_POINT('',#11217) ;
#3174=VERTEX_POINT('',#11219) ;
#3175=VERTEX_POINT('',#11224) ;
#3176=VERTEX_POINT('',#11226) ;
#3177=VERTEX_POINT('',#11231) ;
#3178=VERTEX_POINT('',#11233) ;
#3179=VERTEX_POINT('',#11235) ;
#3180=VERTEX_POINT('',#11237) ;
#3181=VERTEX_POINT('',#11239) ;
#3182=VERTEX_POINT('',#11242) ;
#3183=VERTEX_POINT('',#11244) ;
#3184=VERTEX_POINT('',#11250) ;
#3185=VERTEX_POINT('',#11252) ;
#3186=VERTEX_POINT('',#11258) ;
#3187=VERTEX_POINT('',#11260) ;
#3188=VERTEX_POINT('',#11266) ;
#3189=VERTEX_POINT('',#11268) ;
#3190=VERTEX_POINT('',#11274) ;
#3191=VERTEX_POINT('',#11276) ;
#3192=VERTEX_POINT('',#11282) ;
#3193=VERTEX_POINT('',#11283) ;
#3194=VERTEX_POINT('',#11285) ;
#3195=VERTEX_POINT('',#11287) ;
#3196=VERTEX_POINT('',#11291) ;
#3197=VERTEX_POINT('',#11293) ;
#3198=VERTEX_POINT('',#11297) ;
#3199=VERTEX_POINT('',#11298) ;
#3200=VERTEX_POINT('',#11300) ;
#3201=VERTEX_POINT('',#11302) ;
#3202=VERTEX_POINT('',#11306) ;
#3203=VERTEX_POINT('',#11308) ;
#3204=VERTEX_POINT('',#11312) ;
#3205=VERTEX_POINT('',#11313) ;
#3206=VERTEX_POINT('',#11315) ;
#3207=VERTEX_POINT('',#11317) ;
#3208=VERTEX_POINT('',#11321) ;
#3209=VERTEX_POINT('',#11322) ;
#3210=VERTEX_POINT('',#11324) ;
#3211=VERTEX_POINT('',#11326) ;
#3212=VERTEX_POINT('',#11328) ;
#3213=VERTEX_POINT('',#11331) ;
#3214=VERTEX_POINT('',#11333) ;
#3215=VERTEX_POINT('',#11336) ;
#3216=VERTEX_POINT('',#11343) ;
#3217=VERTEX_POINT('',#11345) ;
#3218=VERTEX_POINT('',#11349) ;
#3219=VERTEX_POINT('',#11358) ;
#3220=VERTEX_POINT('',#11360) ;
#3221=VERTEX_POINT('',#11375) ;
#3222=VERTEX_POINT('',#11377) ;
#3223=VERTEX_POINT('',#11381) ;
#3224=VERTEX_POINT('',#11382) ;
#3225=VERTEX_POINT('',#11384) ;
#3226=VERTEX_POINT('',#11403) ;
#3227=VERTEX_POINT('',#11410) ;
#3228=VERTEX_POINT('',#11425) ;
#3229=VERTEX_POINT('',#11433) ;
#3230=VERTEX_POINT('',#11435) ;
#3231=VERTEX_POINT('',#11441) ;
#3232=VERTEX_POINT('',#11445) ;
#3233=VERTEX_POINT('',#11447) ;
#3234=VERTEX_POINT('',#11451) ;
#3235=VERTEX_POINT('',#11452) ;
#3236=VERTEX_POINT('',#11454) ;
#3237=VERTEX_POINT('',#11473) ;
#3238=VERTEX_POINT('',#11493) ;
#3239=VERTEX_POINT('',#11500) ;
#3240=VERTEX_POINT('',#11502) ;
#3241=VERTEX_POINT('',#11504) ;
#3242=VERTEX_POINT('',#11510) ;
#3243=VERTEX_POINT('',#11512) ;
#3244=VERTEX_POINT('',#11520) ;
#3245=VERTEX_POINT('',#11524) ;
#3246=VERTEX_POINT('',#11528) ;
#3798=EDGE_CURVE('',#3143,#3143,#2637,.F.) ;
#3799=EDGE_CURVE('',#3143,#3144,#1649,.T.) ;
#3800=EDGE_CURVE('',#3144,#3144,#2638,.F.) ;
#3801=EDGE_CURVE('',#3143,#3145,#1650,.T.) ;
#3802=EDGE_CURVE('',#3145,#3145,#2639,.T.) ;
#3803=EDGE_CURVE('',#3146,#3147,#2640,.T.) ;
#3804=EDGE_CURVE('',#3148,#3146,#474,.T.) ;
#3805=EDGE_CURVE('',#3149,#3148,#2641,.T.) ;
#3806=EDGE_CURVE('',#3150,#3149,#475,.T.) ;
#3807=EDGE_CURVE('',#3151,#3150,#2642,.T.) ;
#3808=EDGE_CURVE('',#3152,#3151,#476,.T.) ;
#3809=EDGE_CURVE('',#3147,#3152,#2643,.T.) ;
#3810=EDGE_CURVE('',#3147,#3153,#2644,.T.) ;
#3811=EDGE_CURVE('',#3153,#3153,#2645,.T.) ;
#3812=EDGE_CURVE('',#3153,#3154,#1651,.T.) ;
#3813=EDGE_CURVE('',#3154,#3154,#2646,.T.) ;
#3814=EDGE_CURVE('',#3155,#3155,#2647,.T.) ;
#3815=EDGE_CURVE('',#3155,#3156,#1652,.T.) ;
#3816=EDGE_CURVE('',#3156,#3156,#2648,.T.) ;
#3817=EDGE_CURVE('',#3156,#3157,#1653,.T.) ;
#3818=EDGE_CURVE('',#3157,#3157,#2649,.T.) ;
#3819=EDGE_CURVE('',#3158,#3158,#2650,.T.) ;
#3820=EDGE_CURVE('',#3159,#3159,#2651,.F.) ;
#3821=EDGE_CURVE('',#3159,#3158,#1654,.T.) ;
#3822=EDGE_CURVE('',#3160,#3160,#2652,.T.) ;
#3823=EDGE_CURVE('',#3160,#3161,#2653,.T.) ;
#3824=EDGE_CURVE('',#3161,#3161,#2654,.T.) ;
#3825=EDGE_CURVE('',#3161,#3162,#1655,.T.) ;
#3826=EDGE_CURVE('',#3162,#3162,#2655,.T.) ;
#3827=EDGE_CURVE('',#3162,#3163,#1656,.T.) ;
#3828=EDGE_CURVE('',#3163,#3163,#2656,.T.) ;
#3829=EDGE_CURVE('',#3164,#3164,#2657,.T.) ;
#3830=EDGE_CURVE('',#3164,#3165,#1657,.T.) ;
#3831=EDGE_CURVE('',#3165,#3165,#2658,.T.) ;
#3832=EDGE_CURVE('',#3166,#3166,#2659,.T.) ;
#3833=EDGE_CURVE('',#3166,#3167,#1658,.T.) ;
#3834=EDGE_CURVE('',#3167,#3167,#2660,.T.) ;
#3835=EDGE_CURVE('',#3168,#3168,#2661,.T.) ;
#3836=EDGE_CURVE('',#3168,#3169,#1659,.T.) ;
#3837=EDGE_CURVE('',#3169,#3169,#2662,.T.) ;
#3838=EDGE_CURVE('',#3169,#3170,#1660,.T.) ;
#3839=EDGE_CURVE('',#3170,#3170,#2663,.T.) ;
#3840=EDGE_CURVE('',#3171,#3171,#2664,.T.) ;
#3841=EDGE_CURVE('',#3171,#3172,#1661,.T.) ;
#3842=EDGE_CURVE('',#3172,#3148,#2665,.T.) ;
#3843=EDGE_CURVE('',#3146,#3172,#2666,.T.) ;
#3844=EDGE_CURVE('',#3173,#3173,#2667,.T.) ;
#3845=EDGE_CURVE('',#3173,#3174,#1662,.T.) ;
#3846=EDGE_CURVE('',#3174,#3150,#2668,.T.) ;
#3847=EDGE_CURVE('',#3149,#3174,#2669,.T.) ;
#3848=EDGE_CURVE('',#3175,#3175,#2670,.T.) ;
#3849=EDGE_CURVE('',#3175,#3176,#1663,.T.) ;
#3850=EDGE_CURVE('',#3176,#3152,#2671,.T.) ;
#3851=EDGE_CURVE('',#3151,#3176,#2672,.T.) ;
#3852=EDGE_CURVE('',#3177,#3177,#2673,.T.) ;
#3853=EDGE_CURVE('',#3178,#3178,#2674,.T.) ;
#3854=EDGE_CURVE('',#3179,#3179,#2675,.T.) ;
#3855=EDGE_CURVE('',#3180,#3180,#2676,.T.) ;
#3856=EDGE_CURVE('',#3181,#3181,#2677,.T.) ;
#3857=EDGE_CURVE('',#3182,#3182,#2678,.F.) ;
#3858=EDGE_CURVE('',#3182,#3183,#1664,.T.) ;
#3859=EDGE_CURVE('',#3183,#3183,#2679,.F.) ;
#3860=EDGE_CURVE('',#3182,#3180,#1665,.T.) ;
#3861=EDGE_CURVE('',#3184,#3184,#2680,.F.) ;
#3862=EDGE_CURVE('',#3184,#3185,#1666,.T.) ;
#3863=EDGE_CURVE('',#3185,#3185,#2681,.F.) ;
#3864=EDGE_CURVE('',#3184,#3178,#1667,.T.) ;
#3865=EDGE_CURVE('',#3186,#3186,#2682,.F.) ;
#3866=EDGE_CURVE('',#3186,#3187,#1668,.T.) ;
#3867=EDGE_CURVE('',#3187,#3187,#2683,.F.) ;
#3868=EDGE_CURVE('',#3186,#3181,#1669,.T.) ;
#3869=EDGE_CURVE('',#3188,#3188,#2684,.F.) ;
#3870=EDGE_CURVE('',#3188,#3189,#1670,.T.) ;
#3871=EDGE_CURVE('',#3189,#3189,#2685,.F.) ;
#3872=EDGE_CURVE('',#3188,#3179,#1671,.T.) ;
#3873=EDGE_CURVE('',#3190,#3190,#2686,.F.) ;
#3874=EDGE_CURVE('',#3190,#3191,#1672,.T.) ;
#3875=EDGE_CURVE('',#3191,#3191,#2687,.F.) ;
#3876=EDGE_CURVE('',#3190,#3177,#1673,.T.) ;
#3877=EDGE_CURVE('',#3192,#3193,#2688,.T.) ;
#3878=EDGE_CURVE('',#3192,#3194,#1674,.T.) ;
#3879=EDGE_CURVE('',#3194,#3195,#2689,.T.) ;
#3880=EDGE_CURVE('',#3195,#3193,#1675,.F.) ;
#3881=EDGE_CURVE('',#3196,#3192,#1676,.F.) ;
#3882=EDGE_CURVE('',#3197,#3193,#1677,.F.) ;
#3883=EDGE_CURVE('',#3196,#3197,#2690,.T.) ;
#3884=EDGE_CURVE('',#3198,#3199,#2691,.T.) ;
#3885=EDGE_CURVE('',#3198,#3200,#1678,.T.) ;
#3886=EDGE_CURVE('',#3200,#3201,#2692,.T.) ;
#3887=EDGE_CURVE('',#3201,#3199,#1679,.F.) ;
#3888=EDGE_CURVE('',#3202,#3198,#1680,.F.) ;
#3889=EDGE_CURVE('',#3203,#3199,#1681,.F.) ;
#3890=EDGE_CURVE('',#3202,#3203,#2693,.T.) ;
#3891=EDGE_CURVE('',#3204,#3205,#2694,.T.) ;
#3892=EDGE_CURVE('',#3204,#3206,#1682,.T.) ;
#3893=EDGE_CURVE('',#3206,#3207,#2695,.T.) ;
#3894=EDGE_CURVE('',#3207,#3205,#1683,.F.) ;
#3895=EDGE_CURVE('',#3208,#3209,#1684,.T.) ;
#3896=EDGE_CURVE('',#3209,#3210,#2696,.T.) ;
#3897=EDGE_CURVE('',#3210,#3211,#1685,.T.) ;
#3898=EDGE_CURVE('',#3212,#3211,#2697,.T.) ;
#3899=EDGE_CURVE('',#3212,#3196,#1686,.T.) ;
#3900=EDGE_CURVE('',#3197,#3213,#1687,.T.) ;
#3901=EDGE_CURVE('',#3214,#3213,#2698,.T.) ;
#3902=EDGE_CURVE('',#3214,#3202,#1688,.T.) ;
#3903=EDGE_CURVE('',#3203,#3215,#1689,.T.) ;
#3904=EDGE_CURVE('',#3208,#3215,#2699,.T.) ;
#3905=EDGE_CURVE('',#3209,#3204,#1690,.F.) ;
#3906=EDGE_CURVE('',#3210,#3205,#1691,.F.) ;
#3907=EDGE_CURVE('',#3194,#3216,#1692,.F.) ;
#3908=EDGE_CURVE('',#3217,#3192,#1693,.T.) ;
#3909=EDGE_CURVE('',#3217,#3216,#1694,.F.) ;
#3910=EDGE_CURVE('',#3212,#3218,#477,.T.) ;
#3911=EDGE_CURVE('',#3217,#3218,#187,.F.) ;
#3912=EDGE_CURVE('',#3219,#3216,#2700,.T.) ;
#3913=EDGE_CURVE('',#3218,#3220,#478,.F.) ;
#3914=EDGE_CURVE('',#3220,#3219,#1695,.F.) ;
#3915=EDGE_CURVE('',#3221,#3195,#1696,.F.) ;
#3916=EDGE_CURVE('',#3219,#3222,#2701,.F.) ;
#3917=EDGE_CURVE('',#3221,#3222,#2702,.F.) ;
#3918=EDGE_CURVE('',#3223,#3224,#2703,.T.) ;
#3919=EDGE_CURVE('',#3225,#3223,#479,.F.) ;
#3920=EDGE_CURVE('',#3214,#3225,#480,.T.) ;
#3921=EDGE_CURVE('',#3226,#3213,#481,.F.) ;
#3922=EDGE_CURVE('',#3227,#3226,#482,.T.) ;
#3923=EDGE_CURVE('',#3224,#3227,#2704,.T.) ;
#3924=EDGE_CURVE('',#3193,#3228,#1697,.T.) ;
#3925=EDGE_CURVE('',#3228,#3221,#1698,.F.) ;
#3926=EDGE_CURVE('',#3226,#3228,#188,.T.) ;
#3927=EDGE_CURVE('',#3227,#3222,#1699,.F.) ;
#3928=EDGE_CURVE('',#3200,#3229,#1700,.F.) ;
#3929=EDGE_CURVE('',#3230,#3198,#1701,.T.) ;
#3930=EDGE_CURVE('',#3230,#3229,#1702,.F.) ;
#3931=EDGE_CURVE('',#3230,#3225,#189,.F.) ;
#3932=EDGE_CURVE('',#3231,#3229,#2705,.T.) ;
#3933=EDGE_CURVE('',#3223,#3231,#1703,.F.) ;
#3934=EDGE_CURVE('',#3232,#3201,#1704,.F.) ;
#3935=EDGE_CURVE('',#3231,#3233,#2706,.F.) ;
#3936=EDGE_CURVE('',#3232,#3233,#2707,.F.) ;
#3937=EDGE_CURVE('',#3234,#3235,#2708,.T.) ;
#3938=EDGE_CURVE('',#3236,#3234,#483,.F.) ;
#3939=EDGE_CURVE('',#3208,#3236,#484,.T.) ;
#3940=EDGE_CURVE('',#3237,#3215,#485,.F.) ;
#3941=EDGE_CURVE('',#3235,#3237,#486,.T.) ;
#3942=EDGE_CURVE('',#3199,#3238,#1705,.T.) ;
#3943=EDGE_CURVE('',#3238,#3232,#1706,.F.) ;
#3944=EDGE_CURVE('',#3237,#3238,#190,.T.) ;
#3945=EDGE_CURVE('',#3159,#3224,#1707,.T.) ;
#3946=EDGE_CURVE('',#3220,#3239,#2709,.T.) ;
#3947=EDGE_CURVE('',#3240,#3239,#1708,.F.) ;
#3948=EDGE_CURVE('',#3241,#3240,#2710,.F.) ;
#3949=EDGE_CURVE('',#3241,#3234,#1709,.F.) ;
#3950=EDGE_CURVE('',#3235,#3233,#1710,.T.) ;
#3951=EDGE_CURVE('',#3206,#3242,#1711,.F.) ;
#3952=EDGE_CURVE('',#3243,#3204,#1712,.T.) ;
#3953=EDGE_CURVE('',#3242,#3243,#1713,.F.) ;
#3954=EDGE_CURVE('',#3243,#3236,#191,.F.) ;
#3955=EDGE_CURVE('',#3241,#3242,#2711,.F.) ;
#3956=EDGE_CURVE('',#3244,#3207,#1714,.F.) ;
#3957=EDGE_CURVE('',#3244,#3240,#2712,.F.) ;
#3958=EDGE_CURVE('',#3205,#3245,#1715,.T.) ;
#3959=EDGE_CURVE('',#3244,#3245,#1716,.F.) ;
#3960=EDGE_CURVE('',#3246,#3211,#487,.F.) ;
#3961=EDGE_CURVE('',#3246,#3245,#192,.T.) ;
#3962=EDGE_CURVE('',#3239,#3246,#488,.T.) ;
#4822=ORIENTED_EDGE('',*,*,#3798,.T.) ;
#4823=ORIENTED_EDGE('',*,*,#3799,.T.) ;
#4824=ORIENTED_EDGE('',*,*,#3800,.F.) ;
#4825=ORIENTED_EDGE('',*,*,#3799,.F.) ;
#4826=ORIENTED_EDGE('',*,*,#3798,.F.) ;
#4827=ORIENTED_EDGE('',*,*,#3801,.T.) ;
#4828=ORIENTED_EDGE('',*,*,#3802,.T.) ;
#4829=ORIENTED_EDGE('',*,*,#3801,.F.) ;
#4830=ORIENTED_EDGE('',*,*,#3803,.F.) ;
#4831=ORIENTED_EDGE('',*,*,#3804,.F.) ;
#4832=ORIENTED_EDGE('',*,*,#3805,.F.) ;
#4833=ORIENTED_EDGE('',*,*,#3806,.F.) ;
#4834=ORIENTED_EDGE('',*,*,#3807,.F.) ;
#4835=ORIENTED_EDGE('',*,*,#3808,.F.) ;
#4836=ORIENTED_EDGE('',*,*,#3809,.F.) ;
#4837=ORIENTED_EDGE('',*,*,#3810,.T.) ;
#4838=ORIENTED_EDGE('',*,*,#3811,.T.) ;
#4839=ORIENTED_EDGE('',*,*,#3810,.F.) ;
#4840=ORIENTED_EDGE('',*,*,#3811,.F.) ;
#4841=ORIENTED_EDGE('',*,*,#3812,.T.) ;
#4842=ORIENTED_EDGE('',*,*,#3813,.T.) ;
#4843=ORIENTED_EDGE('',*,*,#3812,.F.) ;
#4844=ORIENTED_EDGE('',*,*,#3814,.T.) ;
#4845=ORIENTED_EDGE('',*,*,#3813,.F.) ;
#4846=ORIENTED_EDGE('',*,*,#3814,.F.) ;
#4847=ORIENTED_EDGE('',*,*,#3815,.T.) ;
#4848=ORIENTED_EDGE('',*,*,#3816,.T.) ;
#4849=ORIENTED_EDGE('',*,*,#3815,.F.) ;
#4850=ORIENTED_EDGE('',*,*,#3816,.F.) ;
#4851=ORIENTED_EDGE('',*,*,#3817,.T.) ;
#4852=ORIENTED_EDGE('',*,*,#3818,.T.) ;
#4853=ORIENTED_EDGE('',*,*,#3817,.F.) ;
#4854=ORIENTED_EDGE('',*,*,#3819,.T.) ;
#4855=ORIENTED_EDGE('',*,*,#3818,.F.) ;
#4856=ORIENTED_EDGE('',*,*,#3820,.T.) ;
#4857=ORIENTED_EDGE('',*,*,#3821,.T.) ;
#4858=ORIENTED_EDGE('',*,*,#3819,.F.) ;
#4859=ORIENTED_EDGE('',*,*,#3821,.F.) ;
#4860=ORIENTED_EDGE('',*,*,#3822,.F.) ;
#4861=ORIENTED_EDGE('',*,*,#3823,.T.) ;
#4862=ORIENTED_EDGE('',*,*,#3824,.T.) ;
#4863=ORIENTED_EDGE('',*,*,#3823,.F.) ;
#4864=ORIENTED_EDGE('',*,*,#3824,.F.) ;
#4865=ORIENTED_EDGE('',*,*,#3825,.T.) ;
#4866=ORIENTED_EDGE('',*,*,#3826,.T.) ;
#4867=ORIENTED_EDGE('',*,*,#3825,.F.) ;
#4868=ORIENTED_EDGE('',*,*,#3826,.F.) ;
#4869=ORIENTED_EDGE('',*,*,#3827,.T.) ;
#4870=ORIENTED_EDGE('',*,*,#3828,.T.) ;
#4871=ORIENTED_EDGE('',*,*,#3827,.F.) ;
#4872=ORIENTED_EDGE('',*,*,#3828,.F.) ;
#4873=ORIENTED_EDGE('',*,*,#3829,.T.) ;
#4874=ORIENTED_EDGE('',*,*,#3829,.F.) ;
#4875=ORIENTED_EDGE('',*,*,#3830,.T.) ;
#4876=ORIENTED_EDGE('',*,*,#3831,.T.) ;
#4877=ORIENTED_EDGE('',*,*,#3830,.F.) ;
#4878=ORIENTED_EDGE('',*,*,#3832,.T.) ;
#4879=ORIENTED_EDGE('',*,*,#3831,.F.) ;
#4880=ORIENTED_EDGE('',*,*,#3832,.F.) ;
#4881=ORIENTED_EDGE('',*,*,#3833,.T.) ;
#4882=ORIENTED_EDGE('',*,*,#3834,.T.) ;
#4883=ORIENTED_EDGE('',*,*,#3833,.F.) ;
#4884=ORIENTED_EDGE('',*,*,#3835,.T.) ;
#4885=ORIENTED_EDGE('',*,*,#3834,.F.) ;
#4886=ORIENTED_EDGE('',*,*,#3835,.F.) ;
#4887=ORIENTED_EDGE('',*,*,#3836,.T.) ;
#4888=ORIENTED_EDGE('',*,*,#3837,.T.) ;
#4889=ORIENTED_EDGE('',*,*,#3836,.F.) ;
#4890=ORIENTED_EDGE('',*,*,#3837,.F.) ;
#4891=ORIENTED_EDGE('',*,*,#3838,.T.) ;
#4892=ORIENTED_EDGE('',*,*,#3839,.T.) ;
#4893=ORIENTED_EDGE('',*,*,#3838,.F.) ;
#4894=ORIENTED_EDGE('',*,*,#3840,.F.) ;
#4895=ORIENTED_EDGE('',*,*,#3841,.T.) ;
#4896=ORIENTED_EDGE('',*,*,#3842,.T.) ;
#4897=ORIENTED_EDGE('',*,*,#3804,.T.) ;
#4898=ORIENTED_EDGE('',*,*,#3843,.T.) ;
#4899=ORIENTED_EDGE('',*,*,#3841,.F.) ;
#4900=ORIENTED_EDGE('',*,*,#3844,.F.) ;
#4901=ORIENTED_EDGE('',*,*,#3845,.T.) ;
#4902=ORIENTED_EDGE('',*,*,#3846,.T.) ;
#4903=ORIENTED_EDGE('',*,*,#3806,.T.) ;
#4904=ORIENTED_EDGE('',*,*,#3847,.T.) ;
#4905=ORIENTED_EDGE('',*,*,#3845,.F.) ;
#4906=ORIENTED_EDGE('',*,*,#3848,.F.) ;
#4907=ORIENTED_EDGE('',*,*,#3849,.T.) ;
#4908=ORIENTED_EDGE('',*,*,#3850,.T.) ;
#4909=ORIENTED_EDGE('',*,*,#3808,.T.) ;
#4910=ORIENTED_EDGE('',*,*,#3851,.T.) ;
#4911=ORIENTED_EDGE('',*,*,#3849,.F.) ;
#4912=ORIENTED_EDGE('',*,*,#3803,.T.) ;
#4913=ORIENTED_EDGE('',*,*,#3809,.T.) ;
#4914=ORIENTED_EDGE('',*,*,#3850,.F.) ;
#4915=ORIENTED_EDGE('',*,*,#3851,.F.) ;
#4916=ORIENTED_EDGE('',*,*,#3807,.T.) ;
#4917=ORIENTED_EDGE('',*,*,#3846,.F.) ;
#4918=ORIENTED_EDGE('',*,*,#3847,.F.) ;
#4919=ORIENTED_EDGE('',*,*,#3805,.T.) ;
#4920=ORIENTED_EDGE('',*,*,#3842,.F.) ;
#4921=ORIENTED_EDGE('',*,*,#3843,.F.) ;
#4922=ORIENTED_EDGE('',*,*,#3802,.F.) ;
#4923=ORIENTED_EDGE('',*,*,#3839,.F.) ;
#4924=ORIENTED_EDGE('',*,*,#3852,.F.) ;
#4925=ORIENTED_EDGE('',*,*,#3853,.F.) ;
#4926=ORIENTED_EDGE('',*,*,#3854,.F.) ;
#4927=ORIENTED_EDGE('',*,*,#3855,.F.) ;
#4928=ORIENTED_EDGE('',*,*,#3856,.F.) ;
#4929=ORIENTED_EDGE('',*,*,#3857,.T.) ;
#4930=ORIENTED_EDGE('',*,*,#3858,.T.) ;
#4931=ORIENTED_EDGE('',*,*,#3859,.F.) ;
#4932=ORIENTED_EDGE('',*,*,#3858,.F.) ;
#4933=ORIENTED_EDGE('',*,*,#3857,.F.) ;
#4934=ORIENTED_EDGE('',*,*,#3860,.T.) ;
#4935=ORIENTED_EDGE('',*,*,#3855,.T.) ;
#4936=ORIENTED_EDGE('',*,*,#3860,.F.) ;
#4937=ORIENTED_EDGE('',*,*,#3861,.T.) ;
#4938=ORIENTED_EDGE('',*,*,#3862,.T.) ;
#4939=ORIENTED_EDGE('',*,*,#3863,.F.) ;
#4940=ORIENTED_EDGE('',*,*,#3862,.F.) ;
#4941=ORIENTED_EDGE('',*,*,#3861,.F.) ;
#4942=ORIENTED_EDGE('',*,*,#3864,.T.) ;
#4943=ORIENTED_EDGE('',*,*,#3853,.T.) ;
#4944=ORIENTED_EDGE('',*,*,#3864,.F.) ;
#4945=ORIENTED_EDGE('',*,*,#3865,.T.) ;
#4946=ORIENTED_EDGE('',*,*,#3866,.T.) ;
#4947=ORIENTED_EDGE('',*,*,#3867,.F.) ;
#4948=ORIENTED_EDGE('',*,*,#3866,.F.) ;
#4949=ORIENTED_EDGE('',*,*,#3865,.F.) ;
#4950=ORIENTED_EDGE('',*,*,#3868,.T.) ;
#4951=ORIENTED_EDGE('',*,*,#3856,.T.) ;
#4952=ORIENTED_EDGE('',*,*,#3868,.F.) ;
#4953=ORIENTED_EDGE('',*,*,#3869,.T.) ;
#4954=ORIENTED_EDGE('',*,*,#3870,.T.) ;
#4955=ORIENTED_EDGE('',*,*,#3871,.F.) ;
#4956=ORIENTED_EDGE('',*,*,#3870,.F.) ;
#4957=ORIENTED_EDGE('',*,*,#3869,.F.) ;
#4958=ORIENTED_EDGE('',*,*,#3872,.T.) ;
#4959=ORIENTED_EDGE('',*,*,#3854,.T.) ;
#4960=ORIENTED_EDGE('',*,*,#3872,.F.) ;
#4961=ORIENTED_EDGE('',*,*,#3873,.T.) ;
#4962=ORIENTED_EDGE('',*,*,#3874,.T.) ;
#4963=ORIENTED_EDGE('',*,*,#3875,.F.) ;
#4964=ORIENTED_EDGE('',*,*,#3874,.F.) ;
#4965=ORIENTED_EDGE('',*,*,#3873,.F.) ;
#4966=ORIENTED_EDGE('',*,*,#3876,.T.) ;
#4967=ORIENTED_EDGE('',*,*,#3852,.T.) ;
#4968=ORIENTED_EDGE('',*,*,#3876,.F.) ;
#4969=ORIENTED_EDGE('',*,*,#3877,.F.) ;
#4970=ORIENTED_EDGE('',*,*,#3878,.T.) ;
#4971=ORIENTED_EDGE('',*,*,#3879,.T.) ;
#4972=ORIENTED_EDGE('',*,*,#3880,.T.) ;
#4973=ORIENTED_EDGE('',*,*,#3881,.T.) ;
#4974=ORIENTED_EDGE('',*,*,#3877,.T.) ;
#4975=ORIENTED_EDGE('',*,*,#3882,.F.) ;
#4976=ORIENTED_EDGE('',*,*,#3883,.F.) ;
#4977=ORIENTED_EDGE('',*,*,#3884,.F.) ;
#4978=ORIENTED_EDGE('',*,*,#3885,.T.) ;
#4979=ORIENTED_EDGE('',*,*,#3886,.T.) ;
#4980=ORIENTED_EDGE('',*,*,#3887,.T.) ;
#4981=ORIENTED_EDGE('',*,*,#3888,.T.) ;
#4982=ORIENTED_EDGE('',*,*,#3884,.T.) ;
#4983=ORIENTED_EDGE('',*,*,#3889,.F.) ;
#4984=ORIENTED_EDGE('',*,*,#3890,.F.) ;
#4985=ORIENTED_EDGE('',*,*,#3891,.F.) ;
#4986=ORIENTED_EDGE('',*,*,#3892,.T.) ;
#4987=ORIENTED_EDGE('',*,*,#3893,.T.) ;
#4988=ORIENTED_EDGE('',*,*,#3894,.T.) ;
#4989=ORIENTED_EDGE('',*,*,#3895,.T.) ;
#4990=ORIENTED_EDGE('',*,*,#3896,.T.) ;
#4991=ORIENTED_EDGE('',*,*,#3897,.T.) ;
#4992=ORIENTED_EDGE('',*,*,#3898,.F.) ;
#4993=ORIENTED_EDGE('',*,*,#3899,.T.) ;
#4994=ORIENTED_EDGE('',*,*,#3883,.T.) ;
#4995=ORIENTED_EDGE('',*,*,#3900,.T.) ;
#4996=ORIENTED_EDGE('',*,*,#3901,.F.) ;
#4997=ORIENTED_EDGE('',*,*,#3902,.T.) ;
#4998=ORIENTED_EDGE('',*,*,#3890,.T.) ;
#4999=ORIENTED_EDGE('',*,*,#3903,.T.) ;
#5000=ORIENTED_EDGE('',*,*,#3904,.F.) ;
#5001=ORIENTED_EDGE('',*,*,#3800,.T.) ;
#5002=ORIENTED_EDGE('',*,*,#3822,.T.) ;
#5003=ORIENTED_EDGE('',*,*,#3875,.T.) ;
#5004=ORIENTED_EDGE('',*,*,#3863,.T.) ;
#5005=ORIENTED_EDGE('',*,*,#3871,.T.) ;
#5006=ORIENTED_EDGE('',*,*,#3859,.T.) ;
#5007=ORIENTED_EDGE('',*,*,#3867,.T.) ;
#5008=ORIENTED_EDGE('',*,*,#3905,.T.) ;
#5009=ORIENTED_EDGE('',*,*,#3891,.T.) ;
#5010=ORIENTED_EDGE('',*,*,#3906,.F.) ;
#5011=ORIENTED_EDGE('',*,*,#3896,.F.) ;
#5012=ORIENTED_EDGE('',*,*,#3907,.F.) ;
#5013=ORIENTED_EDGE('',*,*,#3878,.F.) ;
#5014=ORIENTED_EDGE('',*,*,#3908,.F.) ;
#5015=ORIENTED_EDGE('',*,*,#3909,.T.) ;
#5016=ORIENTED_EDGE('',*,*,#3908,.T.) ;
#5017=ORIENTED_EDGE('',*,*,#3881,.F.) ;
#5018=ORIENTED_EDGE('',*,*,#3899,.F.) ;
#5019=ORIENTED_EDGE('',*,*,#3910,.T.) ;
#5020=ORIENTED_EDGE('',*,*,#3911,.F.) ;
#5021=ORIENTED_EDGE('',*,*,#3912,.T.) ;
#5022=ORIENTED_EDGE('',*,*,#3909,.F.) ;
#5023=ORIENTED_EDGE('',*,*,#3911,.T.) ;
#5024=ORIENTED_EDGE('',*,*,#3913,.T.) ;
#5025=ORIENTED_EDGE('',*,*,#3914,.T.) ;
#5026=ORIENTED_EDGE('',*,*,#3915,.T.) ;
#5027=ORIENTED_EDGE('',*,*,#3879,.F.) ;
#5028=ORIENTED_EDGE('',*,*,#3907,.T.) ;
#5029=ORIENTED_EDGE('',*,*,#3912,.F.) ;
#5030=ORIENTED_EDGE('',*,*,#3916,.T.) ;
#5031=ORIENTED_EDGE('',*,*,#3917,.F.) ;
#5032=ORIENTED_EDGE('',*,*,#3848,.T.) ;
#5033=ORIENTED_EDGE('',*,*,#3918,.F.) ;
#5034=ORIENTED_EDGE('',*,*,#3919,.F.) ;
#5035=ORIENTED_EDGE('',*,*,#3920,.F.) ;
#5036=ORIENTED_EDGE('',*,*,#3901,.T.) ;
#5037=ORIENTED_EDGE('',*,*,#3921,.F.) ;
#5038=ORIENTED_EDGE('',*,*,#3922,.F.) ;
#5039=ORIENTED_EDGE('',*,*,#3923,.F.) ;
#5040=ORIENTED_EDGE('',*,*,#3924,.F.) ;
#5041=ORIENTED_EDGE('',*,*,#3880,.F.) ;
#5042=ORIENTED_EDGE('',*,*,#3915,.F.) ;
#5043=ORIENTED_EDGE('',*,*,#3925,.F.) ;
#5044=ORIENTED_EDGE('',*,*,#3921,.T.) ;
#5045=ORIENTED_EDGE('',*,*,#3900,.F.) ;
#5046=ORIENTED_EDGE('',*,*,#3882,.T.) ;
#5047=ORIENTED_EDGE('',*,*,#3924,.T.) ;
#5048=ORIENTED_EDGE('',*,*,#3926,.F.) ;
#5049=ORIENTED_EDGE('',*,*,#3917,.T.) ;
#5050=ORIENTED_EDGE('',*,*,#3927,.F.) ;
#5051=ORIENTED_EDGE('',*,*,#3922,.T.) ;
#5052=ORIENTED_EDGE('',*,*,#3926,.T.) ;
#5053=ORIENTED_EDGE('',*,*,#3925,.T.) ;
#5054=ORIENTED_EDGE('',*,*,#3928,.F.) ;
#5055=ORIENTED_EDGE('',*,*,#3885,.F.) ;
#5056=ORIENTED_EDGE('',*,*,#3929,.F.) ;
#5057=ORIENTED_EDGE('',*,*,#3930,.T.) ;
#5058=ORIENTED_EDGE('',*,*,#3929,.T.) ;
#5059=ORIENTED_EDGE('',*,*,#3888,.F.) ;
#5060=ORIENTED_EDGE('',*,*,#3902,.F.) ;
#5061=ORIENTED_EDGE('',*,*,#3920,.T.) ;
#5062=ORIENTED_EDGE('',*,*,#3931,.F.) ;
#5063=ORIENTED_EDGE('',*,*,#3932,.T.) ;
#5064=ORIENTED_EDGE('',*,*,#3930,.F.) ;
#5065=ORIENTED_EDGE('',*,*,#3931,.T.) ;
#5066=ORIENTED_EDGE('',*,*,#3919,.T.) ;
#5067=ORIENTED_EDGE('',*,*,#3933,.T.) ;
#5068=ORIENTED_EDGE('',*,*,#3934,.T.) ;
#5069=ORIENTED_EDGE('',*,*,#3886,.F.) ;
#5070=ORIENTED_EDGE('',*,*,#3928,.T.) ;
#5071=ORIENTED_EDGE('',*,*,#3932,.F.) ;
#5072=ORIENTED_EDGE('',*,*,#3935,.T.) ;
#5073=ORIENTED_EDGE('',*,*,#3936,.F.) ;
#5074=ORIENTED_EDGE('',*,*,#3840,.T.) ;
#5075=ORIENTED_EDGE('',*,*,#3937,.F.) ;
#5076=ORIENTED_EDGE('',*,*,#3938,.F.) ;
#5077=ORIENTED_EDGE('',*,*,#3939,.F.) ;
#5078=ORIENTED_EDGE('',*,*,#3904,.T.) ;
#5079=ORIENTED_EDGE('',*,*,#3940,.F.) ;
#5080=ORIENTED_EDGE('',*,*,#3941,.F.) ;
#5081=ORIENTED_EDGE('',*,*,#3942,.F.) ;
#5082=ORIENTED_EDGE('',*,*,#3887,.F.) ;
#5083=ORIENTED_EDGE('',*,*,#3934,.F.) ;
#5084=ORIENTED_EDGE('',*,*,#3943,.F.) ;
#5085=ORIENTED_EDGE('',*,*,#3940,.T.) ;
#5086=ORIENTED_EDGE('',*,*,#3903,.F.) ;
#5087=ORIENTED_EDGE('',*,*,#3889,.T.) ;
#5088=ORIENTED_EDGE('',*,*,#3942,.T.) ;
#5089=ORIENTED_EDGE('',*,*,#3944,.F.) ;
#5090=ORIENTED_EDGE('',*,*,#3820,.F.) ;
#5091=ORIENTED_EDGE('',*,*,#3945,.T.) ;
#5092=ORIENTED_EDGE('',*,*,#3923,.T.) ;
#5093=ORIENTED_EDGE('',*,*,#3927,.T.) ;
#5094=ORIENTED_EDGE('',*,*,#3916,.F.) ;
#5095=ORIENTED_EDGE('',*,*,#3914,.F.) ;
#5096=ORIENTED_EDGE('',*,*,#3946,.T.) ;
#5097=ORIENTED_EDGE('',*,*,#3947,.F.) ;
#5098=ORIENTED_EDGE('',*,*,#3948,.F.) ;
#5099=ORIENTED_EDGE('',*,*,#3949,.T.) ;
#5100=ORIENTED_EDGE('',*,*,#3937,.T.) ;
#5101=ORIENTED_EDGE('',*,*,#3950,.T.) ;
#5102=ORIENTED_EDGE('',*,*,#3935,.F.) ;
#5103=ORIENTED_EDGE('',*,*,#3933,.F.) ;
#5104=ORIENTED_EDGE('',*,*,#3918,.T.) ;
#5105=ORIENTED_EDGE('',*,*,#3945,.F.) ;
#5106=ORIENTED_EDGE('',*,*,#3936,.T.) ;
#5107=ORIENTED_EDGE('',*,*,#3950,.F.) ;
#5108=ORIENTED_EDGE('',*,*,#3941,.T.) ;
#5109=ORIENTED_EDGE('',*,*,#3944,.T.) ;
#5110=ORIENTED_EDGE('',*,*,#3943,.T.) ;
#5111=ORIENTED_EDGE('',*,*,#3951,.F.) ;
#5112=ORIENTED_EDGE('',*,*,#3892,.F.) ;
#5113=ORIENTED_EDGE('',*,*,#3952,.F.) ;
#5114=ORIENTED_EDGE('',*,*,#3953,.F.) ;
#5115=ORIENTED_EDGE('',*,*,#3952,.T.) ;
#5116=ORIENTED_EDGE('',*,*,#3905,.F.) ;
#5117=ORIENTED_EDGE('',*,*,#3895,.F.) ;
#5118=ORIENTED_EDGE('',*,*,#3939,.T.) ;
#5119=ORIENTED_EDGE('',*,*,#3954,.F.) ;
#5120=ORIENTED_EDGE('',*,*,#3954,.T.) ;
#5121=ORIENTED_EDGE('',*,*,#3938,.T.) ;
#5122=ORIENTED_EDGE('',*,*,#3949,.F.) ;
#5123=ORIENTED_EDGE('',*,*,#3955,.T.) ;
#5124=ORIENTED_EDGE('',*,*,#3953,.T.) ;
#5125=ORIENTED_EDGE('',*,*,#3956,.T.) ;
#5126=ORIENTED_EDGE('',*,*,#3893,.F.) ;
#5127=ORIENTED_EDGE('',*,*,#3951,.T.) ;
#5128=ORIENTED_EDGE('',*,*,#3955,.F.) ;
#5129=ORIENTED_EDGE('',*,*,#3948,.T.) ;
#5130=ORIENTED_EDGE('',*,*,#3957,.F.) ;
#5131=ORIENTED_EDGE('',*,*,#3844,.T.) ;
#5132=ORIENTED_EDGE('',*,*,#3958,.F.) ;
#5133=ORIENTED_EDGE('',*,*,#3894,.F.) ;
#5134=ORIENTED_EDGE('',*,*,#3956,.F.) ;
#5135=ORIENTED_EDGE('',*,*,#3959,.T.) ;
#5136=ORIENTED_EDGE('',*,*,#3960,.T.) ;
#5137=ORIENTED_EDGE('',*,*,#3897,.F.) ;
#5138=ORIENTED_EDGE('',*,*,#3906,.T.) ;
#5139=ORIENTED_EDGE('',*,*,#3958,.T.) ;
#5140=ORIENTED_EDGE('',*,*,#3961,.F.) ;
#5141=ORIENTED_EDGE('',*,*,#3946,.F.) ;
#5142=ORIENTED_EDGE('',*,*,#3913,.F.) ;
#5143=ORIENTED_EDGE('',*,*,#3910,.F.) ;
#5144=ORIENTED_EDGE('',*,*,#3898,.T.) ;
#5145=ORIENTED_EDGE('',*,*,#3960,.F.) ;
#5146=ORIENTED_EDGE('',*,*,#3962,.F.) ;
#5147=ORIENTED_EDGE('',*,*,#3962,.T.) ;
#5148=ORIENTED_EDGE('',*,*,#3961,.T.) ;
#5149=ORIENTED_EDGE('',*,*,#3959,.F.) ;
#5150=ORIENTED_EDGE('',*,*,#3957,.T.) ;
#5151=ORIENTED_EDGE('',*,*,#3947,.T.) ;
#6870=CONICAL_SURFACE('',#7572,1.621,1.0471975512) ;
#6871=CONICAL_SURFACE('',#7590,27.5,0.349065850399) ;
#6872=CONICAL_SURFACE('',#7594,28.3,0.785398163397) ;
#6873=CONICAL_SURFACE('',#7602,18.7,0.785398163397) ;
#6874=CONICAL_SURFACE('',#7616,14.,0.523598775598) ;
#6875=CONICAL_SURFACE('',#7636,1.621,1.0471975512) ;
#6876=CONICAL_SURFACE('',#7640,1.621,1.0471975512) ;
#6877=CONICAL_SURFACE('',#7644,1.621,1.0471975512) ;
#6878=CONICAL_SURFACE('',#7648,1.621,1.0471975512) ;
#6879=CONICAL_SURFACE('',#7652,1.621,1.0471975512) ;
#6880=CONICAL_SURFACE('',#7659,1.,0.785398163398) ;
#6881=CONICAL_SURFACE('',#7664,1.,0.785398163398) ;
#6882=CONICAL_SURFACE('',#7674,1.,0.785398163398) ;
#6918=ADVANCED_FACE('',(#668),#6870,.F.) ;
#6919=ADVANCED_FACE('',(#669),#541,.F.) ;
#6920=ADVANCED_FACE('',(#670),#492,.F.) ;
#6921=ADVANCED_FACE('',(#671),#542,.F.) ;
#6922=ADVANCED_FACE('',(#672,#193),#266,.T.) ;
#6923=ADVANCED_FACE('',(#673),#543,.F.) ;
#6924=ADVANCED_FACE('',(#674),#6871,.F.) ;
#6925=ADVANCED_FACE('',(#675,#194),#267,.T.) ;
#6926=ADVANCED_FACE('',(#676),#6872,.T.) ;
#6927=ADVANCED_FACE('',(#677),#493,.F.) ;
#6928=ADVANCED_FACE('',(#678),#544,.T.) ;
#6929=ADVANCED_FACE('',(#679),#6873,.T.) ;
#6930=ADVANCED_FACE('',(#680,#195),#268,.F.) ;
#6931=ADVANCED_FACE('',(#681),#545,.F.) ;
#6932=ADVANCED_FACE('',(#682,#196),#269,.T.) ;
#6933=ADVANCED_FACE('',(#683),#546,.F.) ;
#6934=ADVANCED_FACE('',(#684,#197),#270,.T.) ;
#6935=ADVANCED_FACE('',(#685),#547,.F.) ;
#6936=ADVANCED_FACE('',(#686),#6874,.F.) ;
#6937=ADVANCED_FACE('',(#687),#548,.F.) ;
#6938=ADVANCED_FACE('',(#688),#549,.F.) ;
#6939=ADVANCED_FACE('',(#689),#550,.F.) ;
#6940=ADVANCED_FACE('',(#690,#198,#199,#200,#201,#202,#203,#204),#271,.T.) ;
#6941=ADVANCED_FACE('',(#691),#6875,.F.) ;
#6942=ADVANCED_FACE('',(#692),#551,.F.) ;
#6943=ADVANCED_FACE('',(#693),#6876,.F.) ;
#6944=ADVANCED_FACE('',(#694),#552,.F.) ;
#6945=ADVANCED_FACE('',(#695),#6877,.F.) ;
#6946=ADVANCED_FACE('',(#696),#553,.F.) ;
#6947=ADVANCED_FACE('',(#697),#6878,.F.) ;
#6948=ADVANCED_FACE('',(#698),#554,.F.) ;
#6949=ADVANCED_FACE('',(#699),#6879,.F.) ;
#6950=ADVANCED_FACE('',(#700),#555,.F.) ;
#6951=ADVANCED_FACE('',(#701),#556,.F.) ;
#6952=ADVANCED_FACE('',(#702),#6880,.F.) ;
#6953=ADVANCED_FACE('',(#703),#557,.F.) ;
#6954=ADVANCED_FACE('',(#704),#6881,.F.) ;
#6955=ADVANCED_FACE('',(#705),#558,.F.) ;
#6956=ADVANCED_FACE('',(#706,#205,#206,#207,#208,#209,#210,#211),#272,.F.) ;
#6957=ADVANCED_FACE('',(#707),#6882,.F.) ;
#6958=ADVANCED_FACE('',(#708),#273,.T.) ;
#6959=ADVANCED_FACE('',(#709),#274,.T.) ;
#6960=ADVANCED_FACE('',(#710),#559,.T.) ;
#6961=ADVANCED_FACE('',(#711,#212),#275,.F.) ;
#6962=ADVANCED_FACE('',(#712),#494,.T.) ;
#6963=ADVANCED_FACE('',(#713),#276,.T.) ;
#6964=ADVANCED_FACE('',(#714),#277,.T.) ;
#6965=ADVANCED_FACE('',(#715),#560,.T.) ;
#6966=ADVANCED_FACE('',(#716),#278,.T.) ;
#6967=ADVANCED_FACE('',(#717),#279,.T.) ;
#6968=ADVANCED_FACE('',(#718),#561,.T.) ;
#6969=ADVANCED_FACE('',(#719,#213),#280,.F.) ;
#6970=ADVANCED_FACE('',(#720),#495,.T.) ;
#6971=ADVANCED_FACE('',(#721),#281,.T.) ;
#6972=ADVANCED_FACE('',(#722),#282,.T.) ;
#6973=ADVANCED_FACE('',(#723),#562,.T.) ;
#6974=ADVANCED_FACE('',(#724),#563,.T.) ;
#6975=ADVANCED_FACE('',(#725),#283,.T.) ;
#6976=ADVANCED_FACE('',(#726),#284,.T.) ;
#6977=ADVANCED_FACE('',(#727),#564,.T.) ;
#6978=ADVANCED_FACE('',(#728,#214),#285,.F.) ;
#6979=ADVANCED_FACE('',(#729),#286,.T.) ;
#6980=ADVANCED_FACE('',(#730),#287,.T.) ;
#6981=ADVANCED_FACE('',(#731),#496,.T.) ;
#6982=ADVANCED_FACE('',(#732),#565,.T.) ;
#7372=CLOSED_SHELL('',(#6918,#6919,#6920,#6921,#6922,#6923,#6924,#6925,
#6926,#6927,#6928,#6929,#6930,#6931,#6932,#6933,#6934,#6935,#6936,#6937,
#6938,#6939,#6940,#6941,#6942,#6943,#6944,#6945,#6946,#6947,#6948,#6949,
#6950,#6951,#6952,#6953,#6954,#6955,#6956,#6957,#6958,#6959,#6960,#6961,
#6962,#6963,#6964,#6965,#6966,#6967,#6968,#6969,#6970,#6971,#6972,#6973,
#6974,#6975,#6976,#6977,#6978,#6979,#6980,#6981,#6982)) ;
#7571=AXIS2_PLACEMENT_3D('',#11056,#8569,#8570) ;
#7572=AXIS2_PLACEMENT_3D('',#11057,#8571,#8572) ;
#7573=AXIS2_PLACEMENT_3D('',#11059,#8573,#8574) ;
#7574=AXIS2_PLACEMENT_3D('',#11062,#8576,#8577) ;
#7575=AXIS2_PLACEMENT_3D('',#11063,#8578,#8579) ;
#7576=AXIS2_PLACEMENT_3D('',#11066,#8581,#8582) ;
#7577=AXIS2_PLACEMENT_3D('',#11067,#8583,#8584) ;
#7578=AXIS2_PLACEMENT_3D('',#11070,#8585,#8586) ;
#7579=AXIS2_PLACEMENT_3D('',#11095,#8587,#8588) ;
#7580=AXIS2_PLACEMENT_3D('',#11120,#8589,#8590) ;
#7581=AXIS2_PLACEMENT_3D('',#11144,#8591,#8592) ;
#7582=AXIS2_PLACEMENT_3D('',#11146,#8593,#8594) ;
#7583=AXIS2_PLACEMENT_3D('',#11147,#8595,#8596) ;
#7584=AXIS2_PLACEMENT_3D('',#11148,#8597,#8598) ;
#7585=AXIS2_PLACEMENT_3D('',#11151,#8600,#8601) ;
#7586=AXIS2_PLACEMENT_3D('',#11152,#8602,#8603) ;
#7587=AXIS2_PLACEMENT_3D('',#11154,#8604,#8605) ;
#7588=AXIS2_PLACEMENT_3D('',#11155,#8606,#8607) ;
#7589=AXIS2_PLACEMENT_3D('',#11158,#8609,#8610) ;
#7590=AXIS2_PLACEMENT_3D('',#11159,#8611,#8612) ;
#7591=AXIS2_PLACEMENT_3D('',#11162,#8614,#8615) ;
#7592=AXIS2_PLACEMENT_3D('',#11163,#8616,#8617) ;
#7593=AXIS2_PLACEMENT_3D('',#11165,#8618,#8619) ;
#7594=AXIS2_PLACEMENT_3D('',#11166,#8620,#8621) ;
#7595=AXIS2_PLACEMENT_3D('',#11168,#8622,#8623) ;
#7596=AXIS2_PLACEMENT_3D('',#11170,#8625,#8626) ;
#7597=AXIS2_PLACEMENT_3D('',#11172,#8627,#8628) ;
#7598=AXIS2_PLACEMENT_3D('',#11174,#8629,#8630) ;
#7599=AXIS2_PLACEMENT_3D('',#11175,#8631,#8632) ;
#7600=AXIS2_PLACEMENT_3D('',#11176,#8633,#8634) ;
#7601=AXIS2_PLACEMENT_3D('',#11179,#8636,#8637) ;
#7602=AXIS2_PLACEMENT_3D('',#11180,#8638,#8639) ;
#7603=AXIS2_PLACEMENT_3D('',#11183,#8641,#8642) ;
#7604=AXIS2_PLACEMENT_3D('',#11184,#8643,#8644) ;
#7605=AXIS2_PLACEMENT_3D('',#11186,#8645,#8646) ;
#7606=AXIS2_PLACEMENT_3D('',#11187,#8647,#8648) ;
#7607=AXIS2_PLACEMENT_3D('',#11190,#8650,#8651) ;
#7608=AXIS2_PLACEMENT_3D('',#11191,#8652,#8653) ;
#7609=AXIS2_PLACEMENT_3D('',#11193,#8654,#8655) ;
#7610=AXIS2_PLACEMENT_3D('',#11194,#8656,#8657) ;
#7611=AXIS2_PLACEMENT_3D('',#11197,#8659,#8660) ;
#7612=AXIS2_PLACEMENT_3D('',#11198,#8661,#8662) ;
#7613=AXIS2_PLACEMENT_3D('',#11200,#8663,#8664) ;
#7614=AXIS2_PLACEMENT_3D('',#11201,#8665,#8666) ;
#7615=AXIS2_PLACEMENT_3D('',#11204,#8668,#8669) ;
#7616=AXIS2_PLACEMENT_3D('',#11205,#8670,#8671) ;
#7617=AXIS2_PLACEMENT_3D('',#11208,#8673,#8674) ;
#7618=AXIS2_PLACEMENT_3D('',#11209,#8675,#8676) ;
#7619=AXIS2_PLACEMENT_3D('',#11211,#8677,#8678) ;
#7620=AXIS2_PLACEMENT_3D('',#11214,#8680,#8681) ;
#7621=AXIS2_PLACEMENT_3D('',#11215,#8682,#8683) ;
#7622=AXIS2_PLACEMENT_3D('',#11216,#8684,#8685) ;
#7623=AXIS2_PLACEMENT_3D('',#11218,#8686,#8687) ;
#7624=AXIS2_PLACEMENT_3D('',#11221,#8689,#8690) ;
#7625=AXIS2_PLACEMENT_3D('',#11222,#8691,#8692) ;
#7626=AXIS2_PLACEMENT_3D('',#11223,#8693,#8694) ;
#7627=AXIS2_PLACEMENT_3D('',#11225,#8695,#8696) ;
#7628=AXIS2_PLACEMENT_3D('',#11228,#8698,#8699) ;
#7629=AXIS2_PLACEMENT_3D('',#11229,#8700,#8701) ;
#7630=AXIS2_PLACEMENT_3D('',#11230,#8702,#8703) ;
#7631=AXIS2_PLACEMENT_3D('',#11232,#8704,#8705) ;
#7632=AXIS2_PLACEMENT_3D('',#11234,#8706,#8707) ;
#7633=AXIS2_PLACEMENT_3D('',#11236,#8708,#8709) ;
#7634=AXIS2_PLACEMENT_3D('',#11238,#8710,#8711) ;
#7635=AXIS2_PLACEMENT_3D('',#11240,#8712,#8713) ;
#7636=AXIS2_PLACEMENT_3D('',#11241,#8714,#8715) ;
#7637=AXIS2_PLACEMENT_3D('',#11243,#8716,#8717) ;
#7638=AXIS2_PLACEMENT_3D('',#11246,#8719,#8720) ;
#7639=AXIS2_PLACEMENT_3D('',#11247,#8721,#8722) ;
#7640=AXIS2_PLACEMENT_3D('',#11249,#8724,#8725) ;
#7641=AXIS2_PLACEMENT_3D('',#11251,#8726,#8727) ;
#7642=AXIS2_PLACEMENT_3D('',#11254,#8729,#8730) ;
#7643=AXIS2_PLACEMENT_3D('',#11255,#8731,#8732) ;
#7644=AXIS2_PLACEMENT_3D('',#11257,#8734,#8735) ;
#7645=AXIS2_PLACEMENT_3D('',#11259,#8736,#8737) ;
#7646=AXIS2_PLACEMENT_3D('',#11262,#8739,#8740) ;
#7647=AXIS2_PLACEMENT_3D('',#11263,#8741,#8742) ;
#7648=AXIS2_PLACEMENT_3D('',#11265,#8744,#8745) ;
#7649=AXIS2_PLACEMENT_3D('',#11267,#8746,#8747) ;
#7650=AXIS2_PLACEMENT_3D('',#11270,#8749,#8750) ;
#7651=AXIS2_PLACEMENT_3D('',#11271,#8751,#8752) ;
#7652=AXIS2_PLACEMENT_3D('',#11273,#8754,#8755) ;
#7653=AXIS2_PLACEMENT_3D('',#11275,#8756,#8757) ;
#7654=AXIS2_PLACEMENT_3D('',#11278,#8759,#8760) ;
#7655=AXIS2_PLACEMENT_3D('',#11279,#8761,#8762) ;
#7656=AXIS2_PLACEMENT_3D('',#11281,#8764,#8765) ;
#7657=AXIS2_PLACEMENT_3D('',#11284,#8766,#8767) ;
#7658=AXIS2_PLACEMENT_3D('',#11288,#8769,#8770) ;
#7659=AXIS2_PLACEMENT_3D('',#11290,#8772,#8773) ;
#7660=AXIS2_PLACEMENT_3D('',#11295,#8776,#8777) ;
#7661=AXIS2_PLACEMENT_3D('',#11296,#8778,#8779) ;
#7662=AXIS2_PLACEMENT_3D('',#11299,#8780,#8781) ;
#7663=AXIS2_PLACEMENT_3D('',#11303,#8783,#8784) ;
#7664=AXIS2_PLACEMENT_3D('',#11305,#8786,#8787) ;
#7665=AXIS2_PLACEMENT_3D('',#11310,#8790,#8791) ;
#7666=AXIS2_PLACEMENT_3D('',#11311,#8792,#8793) ;
#7667=AXIS2_PLACEMENT_3D('',#11314,#8794,#8795) ;
#7668=AXIS2_PLACEMENT_3D('',#11318,#8797,#8798) ;
#7669=AXIS2_PLACEMENT_3D('',#11320,#8800,#8801) ;
#7670=AXIS2_PLACEMENT_3D('',#11325,#8803,#8804) ;
#7671=AXIS2_PLACEMENT_3D('',#11329,#8806,#8807) ;
#7672=AXIS2_PLACEMENT_3D('',#11334,#8810,#8811) ;
#7673=AXIS2_PLACEMENT_3D('',#11338,#8814,#8815) ;
#7674=AXIS2_PLACEMENT_3D('',#11339,#8816,#8817) ;
#7675=AXIS2_PLACEMENT_3D('',#11342,#8820,#8821) ;
#7676=AXIS2_PLACEMENT_3D('',#11348,#8825,#8826) ;
#7677=AXIS2_PLACEMENT_3D('',#11356,#8827,#8828) ;
#7678=AXIS2_PLACEMENT_3D('',#11357,#8829,#8830) ;
#7679=AXIS2_PLACEMENT_3D('',#11359,#8831,#8832) ;
#7680=AXIS2_PLACEMENT_3D('',#11374,#8834,#8835) ;
#7681=AXIS2_PLACEMENT_3D('',#11378,#8837,#8838) ;
#7682=AXIS2_PLACEMENT_3D('',#11379,#8839,#8840) ;
#7683=AXIS2_PLACEMENT_3D('',#11380,#8841,#8842) ;
#7684=AXIS2_PLACEMENT_3D('',#11383,#8843,#8844) ;
#7685=AXIS2_PLACEMENT_3D('',#11423,#8845,#8846) ;
#7686=AXIS2_PLACEMENT_3D('',#11424,#8847,#8848) ;
#7687=AXIS2_PLACEMENT_3D('',#11428,#8851,#8852) ;
#7688=AXIS2_PLACEMENT_3D('',#11429,#8853,#8854) ;
#7689=AXIS2_PLACEMENT_3D('',#11430,#8855,#8856) ;
#7690=AXIS2_PLACEMENT_3D('',#11432,#8858,#8859) ;
#7691=AXIS2_PLACEMENT_3D('',#11438,#8863,#8864) ;
#7692=AXIS2_PLACEMENT_3D('',#11439,#8865,#8866) ;
#7693=AXIS2_PLACEMENT_3D('',#11440,#8867,#8868) ;
#7694=AXIS2_PLACEMENT_3D('',#11442,#8869,#8870) ;
#7695=AXIS2_PLACEMENT_3D('',#11444,#8872,#8873) ;
#7696=AXIS2_PLACEMENT_3D('',#11448,#8875,#8876) ;
#7697=AXIS2_PLACEMENT_3D('',#11449,#8877,#8878) ;
#7698=AXIS2_PLACEMENT_3D('',#11450,#8879,#8880) ;
#7699=AXIS2_PLACEMENT_3D('',#11453,#8881,#8882) ;
#7700=AXIS2_PLACEMENT_3D('',#11492,#8883,#8884) ;
#7701=AXIS2_PLACEMENT_3D('',#11496,#8887,#8888) ;
#7702=AXIS2_PLACEMENT_3D('',#11497,#8889,#8890) ;
#7703=AXIS2_PLACEMENT_3D('',#11498,#8891,#8892) ;
#7704=AXIS2_PLACEMENT_3D('',#11501,#8894,#8895) ;
#7705=AXIS2_PLACEMENT_3D('',#11505,#8897,#8898) ;
#7706=AXIS2_PLACEMENT_3D('',#11508,#8901,#8902) ;
#7707=AXIS2_PLACEMENT_3D('',#11509,#8903,#8904) ;
#7708=AXIS2_PLACEMENT_3D('',#11515,#8908,#8909) ;
#7709=AXIS2_PLACEMENT_3D('',#11516,#8910,#8911) ;
#7710=AXIS2_PLACEMENT_3D('',#11517,#8912,#8913) ;
#7711=AXIS2_PLACEMENT_3D('',#11518,#8914,#8915) ;
#7712=AXIS2_PLACEMENT_3D('',#11519,#8916,#8917) ;
#7713=AXIS2_PLACEMENT_3D('',#11522,#8919,#8920) ;
#7714=AXIS2_PLACEMENT_3D('',#11523,#8921,#8922) ;
#7715=AXIS2_PLACEMENT_3D('',#11527,#8925,#8926) ;
#7716=AXIS2_PLACEMENT_3D('',#11535,#8927,#8928) ;
#7717=AXIS2_PLACEMENT_3D('',#11536,#8929,#8930) ;
#7718=AXIS2_PLACEMENT_3D('',#11549,#8931,#8932) ;
#8569=DIRECTION('axis',(0.,0.,1.)) ;
#8570=DIRECTION('refdir',(1.,0.,0.)) ;
#8571=DIRECTION('center_axis',(0.,0.,-1.)) ;
#8572=DIRECTION('ref_axis',(0.877582561890372,0.479425538604204,0.)) ;
#8573=DIRECTION('center_axis',(0.,0.,-1.)) ;
#8574=DIRECTION('ref_axis',(1.,0.,0.)) ;
#8575=DIRECTION('',(-0.760008792516785,-0.415194695655093,-0.499999999997054)) ;
#8576=DIRECTION('center_axis',(0.,0.,-1.)) ;
#8577=DIRECTION('ref_axis',(1.,0.,0.)) ;
#8578=DIRECTION('center_axis',(0.,0.,1.)) ;
#8579=DIRECTION('ref_axis',(0.877582561890372,0.479425538604204,0.)) ;
#8580=DIRECTION('',(0.,0.,1.)) ;
#8581=DIRECTION('center_axis',(0.,0.,1.)) ;
#8582=DIRECTION('ref_axis',(-1.,0.,0.)) ;
#8583=DIRECTION('center_axis',(0.,0.,1.)) ;
#8584=DIRECTION('ref_axis',(-0.479425538604204,0.877582561890372,0.)) ;
#8585=DIRECTION('center_axis',(0.,0.,1.)) ;
#8586=DIRECTION('ref_axis',(-1.,0.,0.)) ;
#8587=DIRECTION('center_axis',(0.,0.,1.)) ;
#8588=DIRECTION('ref_axis',(-1.,0.,0.)) ;
#8589=DIRECTION('center_axis',(0.,0.,1.)) ;
#8590=DIRECTION('ref_axis',(-1.,0.,0.)) ;
#8591=DIRECTION('center_axis',(0.,0.,1.)) ;
#8592=DIRECTION('ref_axis',(-1.,0.,0.)) ;
#8593=DIRECTION('center_axis',(-0.877582561890372,-0.479425538604204,0.)) ;
#8594=DIRECTION('ref_axis',(0.479425538604204,-0.877582561890372,0.)) ;
#8595=DIRECTION('center_axis',(0.,0.,1.)) ;
#8596=DIRECTION('ref_axis',(-1.,0.,0.)) ;
#8597=DIRECTION('center_axis',(0.,0.,1.)) ;
#8598=DIRECTION('ref_axis',(-0.479425538604204,0.877582561890372,0.)) ;
#8599=DIRECTION('',(0.,0.,1.)) ;
#8600=DIRECTION('center_axis',(0.,0.,1.)) ;
#8601=DIRECTION('ref_axis',(-1.,0.,0.)) ;
#8602=DIRECTION('center_axis',(0.,0.,1.)) ;
#8603=DIRECTION('ref_axis',(1.,0.,0.)) ;
#8604=DIRECTION('center_axis',(0.,0.,1.)) ;
#8605=DIRECTION('ref_axis',(-1.,0.,0.)) ;
#8606=DIRECTION('center_axis',(0.,0.,1.)) ;
#8607=DIRECTION('ref_axis',(-0.479425538604204,0.877582561890372,0.)) ;
#8608=DIRECTION('',(0.,0.,1.)) ;
#8609=DIRECTION('center_axis',(0.,0.,1.)) ;
#8610=DIRECTION('ref_axis',(-1.,0.,0.)) ;
#8611=DIRECTION('center_axis',(0.,0.,1.)) ;
#8612=DIRECTION('ref_axis',(-0.479425538604204,0.877582561890372,0.)) ;
#8613=DIRECTION('',(0.163973191427456,-0.300150913597963,0.939692620785862)) ;
#8614=DIRECTION('center_axis',(0.,0.,1.)) ;
#8615=DIRECTION('ref_axis',(-1.,0.,0.)) ;
#8616=DIRECTION('center_axis',(0.,0.,1.)) ;
#8617=DIRECTION('ref_axis',(1.,0.,0.)) ;
#8618=DIRECTION('center_axis',(0.,0.,1.)) ;
#8619=DIRECTION('ref_axis',(-1.,0.,0.)) ;
#8620=DIRECTION('center_axis',(0.,0.,-1.)) ;
#8621=DIRECTION('ref_axis',(-0.479425538604204,0.877582561890372,0.)) ;
#8622=DIRECTION('center_axis',(0.,0.,-1.)) ;
#8623=DIRECTION('ref_axis',(1.,0.,0.)) ;
#8624=DIRECTION('',(-0.339005049420894,0.620544580563467,0.707106781186865)) ;
#8625=DIRECTION('center_axis',(0.,0.,1.)) ;
#8626=DIRECTION('ref_axis',(-0.479425538604204,0.877582561890372,0.)) ;
#8627=DIRECTION('center_axis',(0.,0.,1.)) ;
#8628=DIRECTION('ref_axis',(-1.,0.,0.)) ;
#8629=DIRECTION('center_axis',(-0.877582561890372,-0.479425538604204,0.)) ;
#8630=DIRECTION('ref_axis',(0.479425538604204,-0.877582561890372,0.)) ;
#8631=DIRECTION('center_axis',(0.,0.,1.)) ;
#8632=DIRECTION('ref_axis',(-1.,0.,0.)) ;
#8633=DIRECTION('center_axis',(0.,0.,1.)) ;
#8634=DIRECTION('ref_axis',(-0.479425538604204,0.877582561890372,0.)) ;
#8635=DIRECTION('',(0.,0.,-1.)) ;
#8636=DIRECTION('center_axis',(0.,0.,1.)) ;
#8637=DIRECTION('ref_axis',(-1.,0.,0.)) ;
#8638=DIRECTION('center_axis',(0.,0.,1.)) ;
#8639=DIRECTION('ref_axis',(-0.479425538604204,0.877582561890372,0.)) ;
#8640=DIRECTION('',(-0.339005049420894,0.620544580563467,-0.707106781186865)) ;
#8641=DIRECTION('center_axis',(0.,0.,1.)) ;
#8642=DIRECTION('ref_axis',(-1.,0.,0.)) ;
#8643=DIRECTION('center_axis',(0.,0.,1.)) ;
#8644=DIRECTION('ref_axis',(1.,0.,0.)) ;
#8645=DIRECTION('center_axis',(0.,0.,1.)) ;
#8646=DIRECTION('ref_axis',(-1.,0.,0.)) ;
#8647=DIRECTION('center_axis',(0.,0.,1.)) ;
#8648=DIRECTION('ref_axis',(-0.479425538604204,0.877582561890372,0.)) ;
#8649=DIRECTION('',(0.,0.,1.)) ;
#8650=DIRECTION('center_axis',(0.,0.,1.)) ;
#8651=DIRECTION('ref_axis',(-1.,0.,0.)) ;
#8652=DIRECTION('center_axis',(0.,0.,1.)) ;
#8653=DIRECTION('ref_axis',(1.,0.,0.)) ;
#8654=DIRECTION('center_axis',(0.,0.,1.)) ;
#8655=DIRECTION('ref_axis',(-1.,0.,0.)) ;
#8656=DIRECTION('center_axis',(0.,0.,1.)) ;
#8657=DIRECTION('ref_axis',(-0.479425538604204,0.877582561890372,0.)) ;
#8658=DIRECTION('',(0.,0.,1.)) ;
#8659=DIRECTION('center_axis',(0.,0.,1.)) ;
#8660=DIRECTION('ref_axis',(-1.,0.,0.)) ;
#8661=DIRECTION('center_axis',(0.,0.,1.)) ;
#8662=DIRECTION('ref_axis',(1.,0.,0.)) ;
#8663=DIRECTION('center_axis',(0.,0.,1.)) ;
#8664=DIRECTION('ref_axis',(-1.,0.,0.)) ;
#8665=DIRECTION('center_axis',(0.,0.,1.)) ;
#8666=DIRECTION('ref_axis',(-0.479425538604204,0.877582561890372,0.)) ;
#8667=DIRECTION('',(0.,0.,1.)) ;
#8668=DIRECTION('center_axis',(0.,0.,1.)) ;
#8669=DIRECTION('ref_axis',(-1.,0.,0.)) ;
#8670=DIRECTION('center_axis',(0.,0.,1.)) ;
#8671=DIRECTION('ref_axis',(-0.479425538604204,0.877582561890372,0.)) ;
#8672=DIRECTION('',(0.239712769301978,-0.438791280944959,0.866025403784588)) ;
#8673=DIRECTION('center_axis',(0.,0.,1.)) ;
#8674=DIRECTION('ref_axis',(-1.,0.,0.)) ;
#8675=DIRECTION('center_axis',(0.,0.,1.)) ;
#8676=DIRECTION('ref_axis',(-0.853985976599422,0.520296023213258,0.)) ;
#8677=DIRECTION('center_axis',(0.,0.,1.)) ;
#8678=DIRECTION('ref_axis',(-1.,0.,0.)) ;
#8679=DIRECTION('',(0.,0.,1.)) ;
#8680=DIRECTION('center_axis',(0.,0.,1.)) ;
#8681=DIRECTION('ref_axis',(-1.,0.,0.)) ;
#8682=DIRECTION('center_axis',(0.,0.,1.)) ;
#8683=DIRECTION('ref_axis',(-1.,0.,0.)) ;
#8684=DIRECTION('center_axis',(0.,0.,1.)) ;
#8685=DIRECTION('ref_axis',(0.877582561890372,0.479425538604203,0.)) ;
#8686=DIRECTION('center_axis',(0.,0.,1.)) ;
#8687=DIRECTION('ref_axis',(-1.,0.,0.)) ;
#8688=DIRECTION('',(0.,0.,1.)) ;
#8689=DIRECTION('center_axis',(0.,0.,1.)) ;
#8690=DIRECTION('ref_axis',(-1.,0.,0.)) ;
#8691=DIRECTION('center_axis',(0.,0.,1.)) ;
#8692=DIRECTION('ref_axis',(-1.,0.,0.)) ;
#8693=DIRECTION('center_axis',(0.,0.,1.)) ;
#8694=DIRECTION('ref_axis',(-0.0235965852909093,-0.999721561817394,0.)) ;
#8695=DIRECTION('center_axis',(0.,0.,1.)) ;
#8696=DIRECTION('ref_axis',(-1.,0.,0.)) ;
#8697=DIRECTION('',(0.,0.,1.)) ;
#8698=DIRECTION('center_axis',(0.,0.,1.)) ;
#8699=DIRECTION('ref_axis',(-1.,0.,0.)) ;
#8700=DIRECTION('center_axis',(0.,0.,1.)) ;
#8701=DIRECTION('ref_axis',(-1.,0.,0.)) ;
#8702=DIRECTION('center_axis',(0.,0.,1.)) ;
#8703=DIRECTION('ref_axis',(1.,0.,0.)) ;
#8704=DIRECTION('center_axis',(0.,0.,1.)) ;
#8705=DIRECTION('ref_axis',(-1.,0.,0.)) ;
#8706=DIRECTION('center_axis',(0.,0.,1.)) ;
#8707=DIRECTION('ref_axis',(-1.,0.,0.)) ;
#8708=DIRECTION('center_axis',(0.,0.,1.)) ;
#8709=DIRECTION('ref_axis',(-1.,0.,0.)) ;
#8710=DIRECTION('center_axis',(0.,0.,1.)) ;
#8711=DIRECTION('ref_axis',(-1.,0.,0.)) ;
#8712=DIRECTION('center_axis',(0.,0.,1.)) ;
#8713=DIRECTION('ref_axis',(-1.,0.,0.)) ;
#8714=DIRECTION('center_axis',(0.,0.,-1.)) ;
#8715=DIRECTION('ref_axis',(-0.0235965852909093,-0.999721561817394,0.)) ;
#8716=DIRECTION('center_axis',(0.,0.,-1.)) ;
#8717=DIRECTION('ref_axis',(1.,0.,0.)) ;
#8718=DIRECTION('',(0.0204352423045339,0.865784269246619,-0.499999999997054)) ;
#8719=DIRECTION('center_axis',(0.,0.,-1.)) ;
#8720=DIRECTION('ref_axis',(1.,0.,0.)) ;
#8721=DIRECTION('center_axis',(0.,0.,1.)) ;
#8722=DIRECTION('ref_axis',(-0.0235965852909093,-0.999721561817394,0.)) ;
#8723=DIRECTION('',(0.,0.,1.)) ;
#8724=DIRECTION('center_axis',(0.,0.,-1.)) ;
#8725=DIRECTION('ref_axis',(-0.853985976599423,0.520296023213257,0.)) ;
#8726=DIRECTION('center_axis',(0.,0.,-1.)) ;
#8727=DIRECTION('ref_axis',(1.,0.,0.)) ;
#8728=DIRECTION('',(0.739573550212216,-0.450589573591584,-0.499999999997054)) ;
#8729=DIRECTION('center_axis',(0.,0.,-1.)) ;
#8730=DIRECTION('ref_axis',(1.,0.,0.)) ;
#8731=DIRECTION('center_axis',(0.,0.,1.)) ;
#8732=DIRECTION('ref_axis',(-0.853985976599423,0.520296023213257,0.)) ;
#8733=DIRECTION('',(0.,0.,1.)) ;
#8734=DIRECTION('center_axis',(0.,0.,-1.)) ;
#8735=DIRECTION('ref_axis',(0.853985976599423,-0.520296023213257,0.)) ;
#8736=DIRECTION('center_axis',(0.,0.,-1.)) ;
#8737=DIRECTION('ref_axis',(1.,0.,0.)) ;
#8738=DIRECTION('',(-0.739573550212216,0.450589573591584,-0.499999999997054)) ;
#8739=DIRECTION('center_axis',(0.,0.,-1.)) ;
#8740=DIRECTION('ref_axis',(1.,0.,0.)) ;
#8741=DIRECTION('center_axis',(0.,0.,1.)) ;
#8742=DIRECTION('ref_axis',(0.853985976599423,-0.520296023213257,0.)) ;
#8743=DIRECTION('',(0.,0.,1.)) ;
#8744=DIRECTION('center_axis',(0.,0.,-1.)) ;
#8745=DIRECTION('ref_axis',(-0.877582561890372,-0.479425538604204,0.)) ;
#8746=DIRECTION('center_axis',(0.,0.,-1.)) ;
#8747=DIRECTION('ref_axis',(1.,0.,0.)) ;
#8748=DIRECTION('',(0.760008792516785,0.415194695655093,-0.499999999997054)) ;
#8749=DIRECTION('center_axis',(0.,0.,-1.)) ;
#8750=DIRECTION('ref_axis',(1.,0.,0.)) ;
#8751=DIRECTION('center_axis',(0.,0.,1.)) ;
#8752=DIRECTION('ref_axis',(-0.877582561890372,-0.479425538604204,0.)) ;
#8753=DIRECTION('',(0.,0.,1.)) ;
#8754=DIRECTION('center_axis',(0.,0.,-1.)) ;
#8755=DIRECTION('ref_axis',(0.0235965852909093,0.999721561817394,0.)) ;
#8756=DIRECTION('center_axis',(0.,0.,-1.)) ;
#8757=DIRECTION('ref_axis',(1.,0.,0.)) ;
#8758=DIRECTION('',(-0.0204352423045339,-0.865784269246619,-0.499999999997054)) ;
#8759=DIRECTION('center_axis',(0.,0.,-1.)) ;
#8760=DIRECTION('ref_axis',(1.,0.,0.)) ;
#8761=DIRECTION('center_axis',(0.,0.,1.)) ;
#8762=DIRECTION('ref_axis',(0.0235965852909093,0.999721561817394,0.)) ;
#8763=DIRECTION('',(0.,0.,1.)) ;
#8764=DIRECTION('center_axis',(0.,0.,1.)) ;
#8765=DIRECTION('ref_axis',(-0.86602540378492,0.499999999999167,0.)) ;
#8766=DIRECTION('center_axis',(0.,0.,1.)) ;
#8767=DIRECTION('ref_axis',(-1.,0.,0.)) ;
#8768=DIRECTION('',(0.,0.,1.)) ;
#8769=DIRECTION('center_axis',(0.,0.,1.)) ;
#8770=DIRECTION('ref_axis',(-1.,0.,0.)) ;
#8771=DIRECTION('',(0.,0.,1.)) ;
#8772=DIRECTION('center_axis',(-7.1054273576E-14,-6.12843109593E-13,-1.)) ;
#8773=DIRECTION('ref_axis',(-0.866025403785752,0.499999999997726,-2.44886748830748E-13)) ;
#8774=DIRECTION('',(0.353553390593127,0.612372435696219,-0.707106781186253)) ;
#8775=DIRECTION('',(-0.353553390594877,-0.612372435695786,-0.707106781185753)) ;
#8776=DIRECTION('center_axis',(-2.72397187679E-13,3.24832342227E-13,1.)) ;
#8777=DIRECTION('ref_axis',(-1.,7.58804095478491E-43,-2.72397187679E-13)) ;
#8778=DIRECTION('center_axis',(0.,0.,1.)) ;
#8779=DIRECTION('ref_axis',(0.86602540378492,0.499999999999167,0.)) ;
#8780=DIRECTION('center_axis',(0.,0.,1.)) ;
#8781=DIRECTION('ref_axis',(-1.,0.,0.)) ;
#8782=DIRECTION('',(0.,0.,1.)) ;
#8783=DIRECTION('center_axis',(0.,0.,1.)) ;
#8784=DIRECTION('ref_axis',(-1.,0.,0.)) ;
#8785=DIRECTION('',(0.,0.,1.)) ;
#8786=DIRECTION('center_axis',(-5.15143483426E-13,4.35207425653E-13,-1.)) ;
#8787=DIRECTION('ref_axis',(0.866025403785733,0.499999999997758,-2.28523630416067E-13)) ;
#8788=DIRECTION('',(0.353553390593127,-0.612372435696219,-0.707106781186253)) ;
#8789=DIRECTION('',(-0.353553390592035,0.612372435697061,-0.70710678118607)) ;
#8790=DIRECTION('center_axis',(4.25364358329E-13,7.4868876956E-14,1.)) ;
#8791=DIRECTION('ref_axis',(-1.,-5.20025951221009E-43,4.25364358329E-13)) ;
#8792=DIRECTION('center_axis',(0.,0.,1.)) ;
#8793=DIRECTION('ref_axis',(-5.04646829375071E-16,-1.,0.)) ;
#8794=DIRECTION('center_axis',(0.,0.,1.)) ;
#8795=DIRECTION('ref_axis',(-1.,0.,0.)) ;
#8796=DIRECTION('',(0.,0.,1.)) ;
#8797=DIRECTION('center_axis',(0.,0.,1.)) ;
#8798=DIRECTION('ref_axis',(-1.,0.,0.)) ;
#8799=DIRECTION('',(0.,0.,1.)) ;
#8800=DIRECTION('center_axis',(0.,0.,1.)) ;
#8801=DIRECTION('ref_axis',(1.,0.,0.)) ;
#8802=DIRECTION('',(0.,-1.,0.)) ;
#8803=DIRECTION('center_axis',(0.,0.,1.)) ;
#8804=DIRECTION('ref_axis',(-1.,0.,0.)) ;
#8805=DIRECTION('',(0.,1.,0.)) ;
#8806=DIRECTION('center_axis',(0.,0.,1.)) ;
#8807=DIRECTION('ref_axis',(-1.,0.,0.)) ;
#8808=DIRECTION('',(-0.866025403784329,0.50000000000019,0.)) ;
#8809=DIRECTION('',(0.866025403784329,-0.50000000000019,0.)) ;
#8810=DIRECTION('center_axis',(0.,0.,1.)) ;
#8811=DIRECTION('ref_axis',(-1.,0.,0.)) ;
#8812=DIRECTION('',(0.866025403784329,0.50000000000019,0.)) ;
#8813=DIRECTION('',(-0.866025403784329,-0.50000000000019,0.)) ;
#8814=DIRECTION('center_axis',(0.,0.,1.)) ;
#8815=DIRECTION('ref_axis',(-1.,0.,0.)) ;
#8816=DIRECTION('center_axis',(5.17363929475E-13,1.7763568394E-13,-1.)) ;
#8817=DIRECTION('ref_axis',(2.92127433358158E-14,-1.,-1.77635683939985E-13)) ;
#8818=DIRECTION('',(-0.707106781187048,1.25607396695008E-14,-0.707106781186048)) ;
#8819=DIRECTION('',(0.707106781187048,-1.36912062397009E-12,-0.707106781186048)) ;
#8820=DIRECTION('center_axis',(-0.50000000000019,-0.866025403784329,0.)) ;
#8821=DIRECTION('ref_axis',(-0.866025403784329,0.50000000000019,0.)) ;
#8822=DIRECTION('',(-0.866025403784329,0.50000000000019,0.)) ;
#8823=DIRECTION('',(-0.866025403784329,0.50000000000019,0.)) ;
#8824=DIRECTION('',(0.,0.,-1.)) ;
#8825=DIRECTION('center_axis',(-0.353553390592877,-0.612372435695786,-0.707106781186753)) ;
#8826=DIRECTION('ref_axis',(-0.866025403784504,0.499999999999887,-3.49482655513774E-13)) ;
#8827=DIRECTION('center_axis',(-0.353553390592877,-0.612372435695786,-0.707106781186753)) ;
#8828=DIRECTION('ref_axis',(0.353553390593082,0.612372435696143,-0.707106781186342)) ;
#8829=DIRECTION('center_axis',(0.,0.,-1.)) ;
#8830=DIRECTION('ref_axis',(0.925870094093676,-0.377841989279868,0.)) ;
#8831=DIRECTION('center_axis',(0.,0.,-1.)) ;
#8832=DIRECTION('ref_axis',(1.,0.,0.)) ;
#8833=DIRECTION('',(0.,0.,-1.)) ;
#8834=DIRECTION('center_axis',(0.,0.,1.)) ;
#8835=DIRECTION('ref_axis',(1.,0.,0.)) ;
#8836=DIRECTION('',(0.866025403784329,-0.50000000000019,0.)) ;
#8837=DIRECTION('center_axis',(0.,0.,1.)) ;
#8838=DIRECTION('ref_axis',(-1.,0.,0.)) ;
#8839=DIRECTION('center_axis',(0.,0.,1.)) ;
#8840=DIRECTION('ref_axis',(-1.,0.,0.)) ;
#8841=DIRECTION('center_axis',(0.,0.,1.)) ;
#8842=DIRECTION('ref_axis',(5.9224847248629E-13,-1.,0.)) ;
#8843=DIRECTION('center_axis',(0.,0.,1.)) ;
#8844=DIRECTION('ref_axis',(-1.,0.,0.)) ;
#8845=DIRECTION('center_axis',(0.,0.,1.)) ;
#8846=DIRECTION('ref_axis',(-1.,0.,0.)) ;
#8847=DIRECTION('center_axis',(0.50000000000019,0.866025403784329,0.)) ;
#8848=DIRECTION('ref_axis',(0.866025403784329,-0.50000000000019,0.)) ;
#8849=DIRECTION('',(0.866025403784329,-0.50000000000019,0.)) ;
#8850=DIRECTION('',(0.,0.,-1.)) ;
#8851=DIRECTION('center_axis',(0.353553390592877,0.612372435695786,-0.707106781186753)) ;
#8852=DIRECTION('ref_axis',(0.866025403784504,-0.499999999999887,-3.49482655513774E-13)) ;
#8853=DIRECTION('center_axis',(-0.353553390592877,-0.612372435695786,0.707106781186753)) ;
#8854=DIRECTION('ref_axis',(0.353553390593511,0.612372435695895,0.707106781186342)) ;
#8855=DIRECTION('center_axis',(0.,0.,-1.)) ;
#8856=DIRECTION('ref_axis',(0.50000000000019,0.866025403784329,0.)) ;
#8857=DIRECTION('',(0.,0.,-1.)) ;
#8858=DIRECTION('center_axis',(-0.50000000000019,0.866025403784329,0.)) ;
#8859=DIRECTION('ref_axis',(0.866025403784329,0.50000000000019,0.)) ;
#8860=DIRECTION('',(0.866025403784329,0.50000000000019,0.)) ;
#8861=DIRECTION('',(0.866025403784329,0.50000000000019,0.)) ;
#8862=DIRECTION('',(0.,0.,-1.)) ;
#8863=DIRECTION('center_axis',(-0.353553390592877,0.612372435695786,-0.707106781186753)) ;
#8864=DIRECTION('ref_axis',(0.866025403784504,0.499999999999887,3.49482655513774E-13)) ;
#8865=DIRECTION('center_axis',(-0.353553390592877,0.612372435695786,-0.707106781186753)) ;
#8866=DIRECTION('ref_axis',(0.353553390593082,-0.612372435696143,-0.707106781186342)) ;
#8867=DIRECTION('center_axis',(0.,0.,-1.)) ;
#8868=DIRECTION('ref_axis',(-0.790155808379154,-0.612906027450119,0.)) ;
#8869=DIRECTION('center_axis',(0.,0.,-1.)) ;
#8870=DIRECTION('ref_axis',(1.,0.,0.)) ;
#8871=DIRECTION('',(0.,0.,-1.)) ;
#8872=DIRECTION('center_axis',(0.,0.,1.)) ;
#8873=DIRECTION('ref_axis',(1.,0.,0.)) ;
#8874=DIRECTION('',(-0.866025403784329,-0.50000000000019,0.)) ;
#8875=DIRECTION('center_axis',(0.,0.,1.)) ;
#8876=DIRECTION('ref_axis',(-1.,0.,0.)) ;
#8877=DIRECTION('center_axis',(0.,0.,1.)) ;
#8878=DIRECTION('ref_axis',(-1.,0.,0.)) ;
#8879=DIRECTION('center_axis',(0.,0.,1.)) ;
#8880=DIRECTION('ref_axis',(-0.479425538604204,0.877582561890372,0.)) ;
#8881=DIRECTION('center_axis',(0.,0.,1.)) ;
#8882=DIRECTION('ref_axis',(-1.,0.,0.)) ;
#8883=DIRECTION('center_axis',(0.50000000000019,-0.866025403784329,0.)) ;
#8884=DIRECTION('ref_axis',(-0.866025403784329,-0.50000000000019,0.)) ;
#8885=DIRECTION('',(-0.866025403784329,-0.50000000000019,0.)) ;
#8886=DIRECTION('',(0.,0.,-1.)) ;
#8887=DIRECTION('center_axis',(0.353553390592877,-0.612372435695786,-0.707106781186753)) ;
#8888=DIRECTION('ref_axis',(-0.866025403784504,-0.499999999999887,3.49482655513774E-13)) ;
#8889=DIRECTION('center_axis',(-0.353553390592877,0.612372435695786,0.707106781186753)) ;
#8890=DIRECTION('ref_axis',(0.353553390593511,-0.612372435695895,0.707106781186342)) ;
#8891=DIRECTION('center_axis',(0.,0.,1.)) ;
#8892=DIRECTION('ref_axis',(-0.479425538604204,0.877582561890372,0.)) ;
#8893=DIRECTION('',(0.,0.,-1.)) ;
#8894=DIRECTION('center_axis',(0.,0.,1.)) ;
#8895=DIRECTION('ref_axis',(-1.,0.,0.)) ;
#8896=DIRECTION('',(0.,0.,1.)) ;
#8897=DIRECTION('center_axis',(0.,0.,1.)) ;
#8898=DIRECTION('ref_axis',(-1.,0.,0.)) ;
#8899=DIRECTION('',(0.,0.,1.)) ;
#8900=DIRECTION('',(0.,0.,1.)) ;
#8901=DIRECTION('center_axis',(0.,0.,-1.)) ;
#8902=DIRECTION('ref_axis',(0.50000000000019,-0.866025403784329,0.)) ;
#8903=DIRECTION('center_axis',(1.,0.,0.)) ;
#8904=DIRECTION('ref_axis',(0.,-1.,0.)) ;
#8905=DIRECTION('',(0.,-1.,0.)) ;
#8906=DIRECTION('',(0.,-1.,0.)) ;
#8907=DIRECTION('',(0.,0.,1.)) ;
#8908=DIRECTION('center_axis',(0.707106781186548,0.,-0.707106781186548)) ;
#8909=DIRECTION('ref_axis',(0.,-1.,0.)) ;
#8910=DIRECTION('center_axis',(0.707106781186548,0.,-0.707106781186548)) ;
#8911=DIRECTION('ref_axis',(0.707106781186547,0.,0.707106781186547)) ;
#8912=DIRECTION('center_axis',(0.,0.,1.)) ;
#8913=DIRECTION('ref_axis',(1.,0.,0.)) ;
#8914=DIRECTION('center_axis',(0.,0.,1.)) ;
#8915=DIRECTION('ref_axis',(-1.,0.,0.)) ;
#8916=DIRECTION('center_axis',(0.,0.,1.)) ;
#8917=DIRECTION('ref_axis',(1.,0.,0.)) ;
#8918=DIRECTION('',(0.,1.,0.)) ;
#8919=DIRECTION('center_axis',(0.,0.,1.)) ;
#8920=DIRECTION('ref_axis',(-1.,0.,0.)) ;
#8921=DIRECTION('center_axis',(-1.,1.26882631386E-16,0.)) ;
#8922=DIRECTION('ref_axis',(1.26882631386E-16,1.,0.)) ;
#8923=DIRECTION('',(1.62020506058E-16,1.,0.)) ;
#8924=DIRECTION('',(0.,0.,1.)) ;
#8925=DIRECTION('center_axis',(-0.707106781186548,8.84255722483432E-17,
-0.707106781186548)) ;
#8926=DIRECTION('ref_axis',(1.25052643534105E-16,1.,1.04175887789636E-28)) ;
#8927=DIRECTION('center_axis',(0.707106781186548,-8.84255722483432E-17,
0.707106781186548)) ;
#8928=DIRECTION('ref_axis',(0.707106781186547,-2.4532694666934E-17,-0.707106781186547)) ;
#8929=DIRECTION('center_axis',(0.,0.,1.)) ;
#8930=DIRECTION('ref_axis',(-0.479425538604204,0.877582561890372,0.)) ;
#8931=DIRECTION('center_axis',(0.,0.,1.)) ;
#8932=DIRECTION('ref_axis',(0.135714285714047,0.990748016729343,0.)) ;
#11056=CARTESIAN_POINT('',(0.,0.,0.)) ;
#11057=CARTESIAN_POINT('Origin',(22.5,0.,6.21881575202)) ;
#11058=CARTESIAN_POINT('',(21.0774386671757,-0.777148798077412,6.21881575202)) ;
#11059=CARTESIAN_POINT('Origin',(22.5,0.,6.21881575202)) ;
#11060=CARTESIAN_POINT('',(20.7448348762197,-0.958851077208169,5.99999999999914)) ;
#11061=CARTESIAN_POINT('',(21.0774386671757,-0.777148798077415,6.21881575202)) ;
#11062=CARTESIAN_POINT('Origin',(22.5,0.,6.)) ;
#11063=CARTESIAN_POINT('Origin',(22.5,0.,6.1)) ;
#11064=CARTESIAN_POINT('',(21.0774386672,-0.777148798077,11.)) ;
#11065=CARTESIAN_POINT('',(21.0774386671757,-0.777148798077415,6.1)) ;
#11066=CARTESIAN_POINT('Origin',(22.5,0.,11.)) ;
#11067=CARTESIAN_POINT('Origin',(0.,0.,11.5)) ;
#11068=CARTESIAN_POINT('',(-22.6577023948,-13.7433082695,11.)) ;
#11069=CARTESIAN_POINT('',(12.7047767730114,-23.2559378900949,11.)) ;
#11070=CARTESIAN_POINT('Origin',(0.,0.,11.)) ;
#11071=CARTESIAN_POINT('',(-23.2309052908,-12.7504917305,11.)) ;
#11072=CARTESIAN_POINT('Ctrl Pts',(-23.2309052907855,-12.7504917304977,
11.)) ;
#11073=CARTESIAN_POINT('Ctrl Pts',(-23.2177559943721,-12.8334463301629,
10.9999999999989)) ;
#11074=CARTESIAN_POINT('Ctrl Pts',(-23.1976386279022,-12.9181615098257,
11.0023979762017)) ;
#11075=CARTESIAN_POINT('Ctrl Pts',(-23.1423592549325,-13.0849091600432,
11.0070492874094)) ;
#11076=CARTESIAN_POINT('Ctrl Pts',(-23.1087958484009,-13.1642287206961,
11.0091389064929)) ;
#11077=CARTESIAN_POINT('Ctrl Pts',(-23.062837122101,-13.2522341930896,11.0099336516974)) ;
#11078=CARTESIAN_POINT('Ctrl Pts',(-23.0566380161127,-13.2637587597182,
11.0100089133404)) ;
#11079=CARTESIAN_POINT('Ctrl Pts',(-23.0474708103016,-13.2803100920526,
11.0100733355158)) ;
#11080=CARTESIAN_POINT('Ctrl Pts',(-23.0446206015924,-13.28539061731,11.0100871242746)) ;
#11081=CARTESIAN_POINT('Ctrl Pts',(-23.0396068424599,-13.2942141484541,
11.010100495387)) ;
#11082=CARTESIAN_POINT('Ctrl Pts',(-23.0374567977516,-13.2979625812012,
11.0101028410784)) ;
#11083=CARTESIAN_POINT('Ctrl Pts',(-23.0332806953934,-13.3051752649317,
11.0101008710609)) ;
#11084=CARTESIAN_POINT('Ctrl Pts',(-23.0312570240619,-13.3086403575065,
11.0100970327484)) ;
#11085=CARTESIAN_POINT('Ctrl Pts',(-23.0264410266058,-13.31681574998,11.0100811037365)) ;
#11086=CARTESIAN_POINT('Ctrl Pts',(-23.0236367738899,-13.3215208217782,
11.0100665328614)) ;
#11087=CARTESIAN_POINT('Ctrl Pts',(-23.0137708517244,-13.3378821306485,
11.0099969967108)) ;
#11088=CARTESIAN_POINT('Ctrl Pts',(-23.0065803507821,-13.3494697625835,
11.0099141991786)) ;
#11089=CARTESIAN_POINT('Ctrl Pts',(-22.9190880086091,-13.486513956227,11.0085451648483)) ;
#11090=CARTESIAN_POINT('Ctrl Pts',(-22.8279936863588,-13.5908345387433,
11.0032435600432)) ;
#11091=CARTESIAN_POINT('Ctrl Pts',(-22.7093329565058,-13.7001447600221,
11.0003818328419)) ;
#11092=CARTESIAN_POINT('Ctrl Pts',(-22.683635473578,-13.7223027342348,10.9999999999999)) ;
#11093=CARTESIAN_POINT('Ctrl Pts',(-22.6577023947726,-13.7433082694662,
11.)) ;
#11094=CARTESIAN_POINT('',(-0.573202896015,26.4938,11.)) ;
#11095=CARTESIAN_POINT('Origin',(0.,0.,11.)) ;
#11096=CARTESIAN_POINT('',(0.573202896015,26.4938,11.)) ;
#11097=CARTESIAN_POINT('Ctrl Pts',(0.573202896015001,26.4938,11.)) ;
#11098=CARTESIAN_POINT('Ctrl Pts',(0.494787457144988,26.5238896750921,11.)) ;
#11099=CARTESIAN_POINT('Ctrl Pts',(0.411363276244769,26.5488251144995,11.002397976203)) ;
#11100=CARTESIAN_POINT('Ctrl Pts',(0.23931588866044,26.5843255983089,11.0070492874111)) ;
#11101=CARTESIAN_POINT('Ctrl Pts',(0.153841430852333,26.5949186159412,11.0091389064948)) ;
#11102=CARTESIAN_POINT('Ctrl Pts',(0.0546470929391302,26.5991199276366,
11.0099336516993)) ;
#11103=CARTESIAN_POINT('Ctrl Pts',(0.0415669724770221,26.5995136276842,
11.0100089133423)) ;
#11104=CARTESIAN_POINT('Ctrl Pts',(0.0226494953019741,26.5998502607374,
11.0100733355177)) ;
#11105=CARTESIAN_POINT('Ctrl Pts',(0.0168245270108277,26.5999221702178,
11.0100871242765)) ;
#11106=CARTESIAN_POINT('Ctrl Pts',(0.00667624532263877,26.5999918930126,
11.010100495389)) ;
#11107=CARTESIAN_POINT('Ctrl Pts',(0.00235498498562617,26.6000041160495,
11.0101028410803)) ;
#11108=CARTESIAN_POINT('Ctrl Pts',(-0.0059794335320967,26.5999938471837,
11.0101008710628)) ;
#11109=CARTESIAN_POINT('Ctrl Pts',(-0.00999212739330856,26.5999738426891,
11.0100970327503)) ;
#11110=CARTESIAN_POINT('Ctrl Pts',(-0.0194802236908106,26.5998907627844,
11.0100811037385)) ;
#11111=CARTESIAN_POINT('Ctrl Pts',(-0.0249570617525531,26.5998147445928,
11.0100665328633)) ;
#11112=CARTESIAN_POINT('Ctrl Pts',(-0.0440593319568355,26.5994512598009,
11.0099969967128)) ;
#11113=CARTESIAN_POINT('Ctrl Pts',(-0.0576897660537948,26.5990179192864,
11.0099141991805)) ;
#11114=CARTESIAN_POINT('Ctrl Pts',(-0.220119690294974,26.5917694251488,
11.0085451648498)) ;
#11115=CARTESIAN_POINT('Ctrl Pts',(-0.356011126032057,26.565039719192,11.0032435600431)) ;
#11116=CARTESIAN_POINT('Ctrl Pts',(-0.510006919478298,26.5169316233422,
11.0003818328418)) ;
#11117=CARTESIAN_POINT('Ctrl Pts',(-0.542045029494008,26.5057559374237,
11.)) ;
#11118=CARTESIAN_POINT('Ctrl Pts',(-0.573202896015002,26.4938,11.)) ;
#11119=CARTESIAN_POINT('',(23.2309052908,-12.7504917305,11.)) ;
#11120=CARTESIAN_POINT('Origin',(0.,0.,11.)) ;
#11121=CARTESIAN_POINT('',(22.6577023948,-13.7433082695,11.)) ;
#11122=CARTESIAN_POINT('Ctrl Pts',(22.6577023947726,-13.7433082694662,11.)) ;
#11123=CARTESIAN_POINT('Ctrl Pts',(22.7229685372257,-13.690443344904,10.9999999999996)) ;
#11124=CARTESIAN_POINT('Ctrl Pts',(22.786275351654,-13.6306636046609,11.0023979762021)) ;
#11125=CARTESIAN_POINT('Ctrl Pts',(22.9030433662692,-13.4994164382662,11.0070492874094)) ;
#11126=CARTESIAN_POINT('Ctrl Pts',(22.9549544175459,-13.4306898952458,11.0091389064929)) ;
#11127=CARTESIAN_POINT('Ctrl Pts',(23.0081900291609,-13.3468857345477,11.0099336516974)) ;
#11128=CARTESIAN_POINT('Ctrl Pts',(23.0150710436348,-13.3357548679667,11.0100089133404)) ;
#11129=CARTESIAN_POINT('Ctrl Pts',(23.0248213149975,-13.3195401686852,11.0100733355158)) ;
#11130=CARTESIAN_POINT('Ctrl Pts',(23.0277960745803,-13.3145315529084,11.0100871242746)) ;
#11131=CARTESIAN_POINT('Ctrl Pts',(23.0329305971365,-13.3057777445581,11.010100495387)) ;
#11132=CARTESIAN_POINT('Ctrl Pts',(23.0351018127654,-13.3020415348484,11.0101028410783)) ;
#11133=CARTESIAN_POINT('Ctrl Pts',(23.0392601289253,-13.294818582254,11.0101008710609)) ;
#11134=CARTESIAN_POINT('Ctrl Pts',(23.0412491514551,-13.2913334851858,11.0100970327484)) ;
#11135=CARTESIAN_POINT('Ctrl Pts',(23.0459212502966,-13.2830750128048,11.0100811037365)) ;
#11136=CARTESIAN_POINT('Ctrl Pts',(23.0485938356427,-13.2782939228147,11.0100665328614)) ;
#11137=CARTESIAN_POINT('Ctrl Pts',(23.0578301836804,-13.2615691291531,11.0099969967108)) ;
#11138=CARTESIAN_POINT('Ctrl Pts',(23.0642701168348,-13.2495481567036,11.0099141991786)) ;
#11139=CARTESIAN_POINT('Ctrl Pts',(23.1392076988851,-13.1052554689228,11.0085451648482)) ;
#11140=CARTESIAN_POINT('Ctrl Pts',(23.1840048123566,-12.9742051804553,11.0032435600432)) ;
#11141=CARTESIAN_POINT('Ctrl Pts',(23.2193398759538,-12.8167868633182,11.0003818328416)) ;
#11142=CARTESIAN_POINT('Ctrl Pts',(23.2256805030566,-12.78345320317,10.9999999999995)) ;
#11143=CARTESIAN_POINT('Ctrl Pts',(23.2309052907855,-12.7504917304977,11.)) ;
#11144=CARTESIAN_POINT('Origin',(0.,0.,11.)) ;
#11145=CARTESIAN_POINT('',(12.9444895423,-23.694729171,11.5)) ;
#11146=CARTESIAN_POINT('Origin',(12.7047767730114,-23.2559378900949,11.5)) ;
#11147=CARTESIAN_POINT('Origin',(0.,0.,11.5)) ;
#11148=CARTESIAN_POINT('Origin',(0.,0.,10.5000000001)) ;
#11149=CARTESIAN_POINT('',(12.9444895423135,-23.6947291710401,19.5)) ;
#11150=CARTESIAN_POINT('',(12.9444895423135,-23.69472917104,10.5000000001)) ;
#11151=CARTESIAN_POINT('Origin',(0.,0.,19.5)) ;
#11152=CARTESIAN_POINT('Origin',(0.,27.5,19.5)) ;
#11153=CARTESIAN_POINT('',(13.1842023116,-24.133520452,19.5)) ;
#11154=CARTESIAN_POINT('Origin',(0.,0.,19.5)) ;
#11155=CARTESIAN_POINT('Origin',(0.,0.,10.5000000001)) ;
#11156=CARTESIAN_POINT('',(13.1842023116,-24.133520452,19.6262612903)) ;
#11157=CARTESIAN_POINT('',(13.1842023116156,-24.1335204519852,10.5000000001)) ;
#11158=CARTESIAN_POINT('Origin',(0.,0.,19.6262612903)) ;
#11159=CARTESIAN_POINT('Origin',(0.,0.,19.6262612903)) ;
#11160=CARTESIAN_POINT('',(13.4239150809,-24.5723117329,21.)) ;
#11161=CARTESIAN_POINT('',(13.1842023116156,-24.1335204519852,19.6262612903)) ;
#11162=CARTESIAN_POINT('Origin',(0.,0.,21.)) ;
#11163=CARTESIAN_POINT('Origin',(0.,28.3,21.)) ;
#11164=CARTESIAN_POINT('',(13.5677427425,-24.8355865015,21.)) ;
#11165=CARTESIAN_POINT('Origin',(0.,0.,21.)) ;
#11166=CARTESIAN_POINT('Origin',(0.,0.,21.)) ;
#11167=CARTESIAN_POINT('',(13.6636278502,-25.0111030139,20.8)) ;
#11168=CARTESIAN_POINT('Origin',(0.,0.,20.8)) ;
#11169=CARTESIAN_POINT('',(13.567742742499,-24.8355865014975,21.)) ;
#11170=CARTESIAN_POINT('Origin',(0.,0.,5.6)) ;
#11171=CARTESIAN_POINT('',(9.30085544892155,-17.0251017006732,6.)) ;
#11172=CARTESIAN_POINT('Origin',(0.,0.,6.)) ;
#11173=CARTESIAN_POINT('',(9.10908523347987,-16.6740686759171,5.6)) ;
#11174=CARTESIAN_POINT('Origin',(9.30085544892156,-17.0251017006732,5.6)) ;
#11175=CARTESIAN_POINT('Origin',(0.,0.,5.6)) ;
#11176=CARTESIAN_POINT('Origin',(0.,0.,10.5000000001)) ;
#11177=CARTESIAN_POINT('',(9.10908523347987,-16.6740686759171,0.3)) ;
#11178=CARTESIAN_POINT('',(9.10908523347988,-16.6740686759171,10.5000000001)) ;
#11179=CARTESIAN_POINT('Origin',(0.,0.,0.3)) ;
#11180=CARTESIAN_POINT('Origin',(0.,0.,0.)) ;
#11181=CARTESIAN_POINT('',(8.96525757189861,-16.41079390735,-5.09417592659295E-15)) ;
#11182=CARTESIAN_POINT('',(8.96525757189862,-16.41079390735,0.)) ;
#11183=CARTESIAN_POINT('Origin',(0.,0.,0.)) ;
#11184=CARTESIAN_POINT('Origin',(0.,7.8,0.)) ;
#11185=CARTESIAN_POINT('',(3.73951920111279,-6.8451439827449,0.)) ;
#11186=CARTESIAN_POINT('Origin',(0.,0.,0.)) ;
#11187=CARTESIAN_POINT('Origin',(0.,0.,10.5000000001)) ;
#11188=CARTESIAN_POINT('',(3.73951920111279,-6.8451439827449,2.8)) ;
#11189=CARTESIAN_POINT('',(3.73951920111279,-6.8451439827449,10.5000000001)) ;
#11190=CARTESIAN_POINT('Origin',(0.,0.,2.8)) ;
#11191=CARTESIAN_POINT('Origin',(0.,12.5,2.8)) ;
#11192=CARTESIAN_POINT('',(5.99281923255,-10.9697820236,2.8)) ;
#11193=CARTESIAN_POINT('Origin',(0.,0.,2.8)) ;
#11194=CARTESIAN_POINT('Origin',(0.,0.,10.5000000001)) ;
#11195=CARTESIAN_POINT('',(5.99281923255,-10.9697820236,3.)) ;
#11196=CARTESIAN_POINT('',(5.99281923255255,-10.9697820236297,10.5000000001)) ;
#11197=CARTESIAN_POINT('Origin',(0.,0.,3.)) ;
#11198=CARTESIAN_POINT('Origin',(0.,14.,3.)) ;
#11199=CARTESIAN_POINT('',(6.71195754046,-12.2861558665,3.)) ;
#11200=CARTESIAN_POINT('Origin',(0.,0.,3.)) ;
#11201=CARTESIAN_POINT('Origin',(0.,0.,10.5000000001)) ;
#11202=CARTESIAN_POINT('',(6.71195754046,-12.2861558665,10.)) ;
#11203=CARTESIAN_POINT('',(6.71195754045886,-12.2861558664652,10.5000000001)) ;
#11204=CARTESIAN_POINT('Origin',(0.,0.,10.)) ;
#11205=CARTESIAN_POINT('Origin',(0.,0.,10.)) ;
#11206=CARTESIAN_POINT('',(6.98875400423,-12.7928283948,11.)) ;
#11207=CARTESIAN_POINT('',(6.71195754045886,-12.2861558664652,10.)) ;
#11208=CARTESIAN_POINT('Origin',(0.,0.,11.)) ;
#11209=CARTESIAN_POINT('Origin',(-21.6506350946,-12.5,6.1)) ;
#11210=CARTESIAN_POINT('',(-20.2842575321,-13.3324736371,8.8)) ;
#11211=CARTESIAN_POINT('Origin',(-21.6506350946,-12.5,8.8)) ;
#11212=CARTESIAN_POINT('',(-20.2842575320409,-13.3324736371412,11.)) ;
#11213=CARTESIAN_POINT('',(-20.2842575320409,-13.3324736371412,6.1)) ;
#11214=CARTESIAN_POINT('Origin',(-21.6506350946,-12.5,11.)) ;
#11215=CARTESIAN_POINT('Origin',(-21.6506350946,-12.5,11.)) ;
#11216=CARTESIAN_POINT('Origin',(0.,25.,6.1)) ;
#11217=CARTESIAN_POINT('',(-1.40413209902,24.2329191382,8.8)) ;
#11218=CARTESIAN_POINT('Origin',(0.,25.,8.8)) ;
#11219=CARTESIAN_POINT('',(-1.4041320990246,24.2329191382333,11.)) ;
#11220=CARTESIAN_POINT('',(-1.4041320990246,24.2329191382333,6.1)) ;
#11221=CARTESIAN_POINT('Origin',(0.,25.,11.)) ;
#11222=CARTESIAN_POINT('Origin',(0.,25.,11.)) ;
#11223=CARTESIAN_POINT('Origin',(21.6506350946,-12.5,6.1)) ;
#11224=CARTESIAN_POINT('',(21.6883896311,-10.9004455011,8.8)) ;
#11225=CARTESIAN_POINT('Origin',(21.6506350946,-12.5,8.8)) ;
#11226=CARTESIAN_POINT('',(21.6883896310655,-10.9004455010922,11.)) ;
#11227=CARTESIAN_POINT('',(21.6883896310655,-10.9004455010922,6.1)) ;
#11228=CARTESIAN_POINT('Origin',(21.6506350946,-12.5,11.)) ;
#11229=CARTESIAN_POINT('Origin',(21.6506350946,-12.5,11.)) ;
#11230=CARTESIAN_POINT('Origin',(0.,26.5,11.)) ;
#11231=CARTESIAN_POINT('',(11.2117499352,17.8650229334,11.)) ;
#11232=CARTESIAN_POINT('Origin',(11.25,19.4855715851,11.)) ;
#11233=CARTESIAN_POINT('',(-9.86568873193,18.6421717315,11.)) ;
#11234=CARTESIAN_POINT('Origin',(-11.25,19.4855715851,11.)) ;
#11235=CARTESIAN_POINT('',(-21.0774386672,0.777148798077,11.)) ;
#11236=CARTESIAN_POINT('Origin',(-22.5,-7.1054273576E-15,11.)) ;
#11237=CARTESIAN_POINT('',(-11.2117499352,-17.8650229334,11.)) ;
#11238=CARTESIAN_POINT('Origin',(-11.25,-19.4855715851,11.)) ;
#11239=CARTESIAN_POINT('',(9.86568873193,-18.6421717315,11.)) ;
#11240=CARTESIAN_POINT('Origin',(11.25,-19.4855715851,11.)) ;
#11241=CARTESIAN_POINT('Origin',(-11.25,-19.4855715851,6.21881575202)) ;
#11242=CARTESIAN_POINT('',(-11.2117499352434,-17.865022933394,6.21881575202)) ;
#11243=CARTESIAN_POINT('Origin',(-11.25,-19.4855715851,6.21881575202)) ;
#11244=CARTESIAN_POINT('',(-11.2028068294182,-17.4861284614657,5.99999999999914)) ;
#11245=CARTESIAN_POINT('',(-11.2117499352434,-17.865022933394,6.21881575202)) ;
#11246=CARTESIAN_POINT('Origin',(-11.25,-19.4855715851,6.)) ;
#11247=CARTESIAN_POINT('Origin',(-11.25,-19.4855715851,6.1)) ;
#11248=CARTESIAN_POINT('',(-11.2117499352434,-17.865022933394,6.1)) ;
#11249=CARTESIAN_POINT('Origin',(-11.25,19.4855715851,6.21881575202)) ;
#11250=CARTESIAN_POINT('',(-9.86568873193234,18.6421717314713,6.21881575202)) ;
#11251=CARTESIAN_POINT('Origin',(-11.25,19.4855715851,6.21881575202)) ;
#11252=CARTESIAN_POINT('',(-9.54202804680158,18.4449795386737,5.99999999999914)) ;
#11253=CARTESIAN_POINT('',(-9.86568873193234,18.6421717314713,6.21881575202)) ;
#11254=CARTESIAN_POINT('Origin',(-11.25,19.4855715851,6.)) ;
#11255=CARTESIAN_POINT('Origin',(-11.25,19.4855715851,6.1)) ;
#11256=CARTESIAN_POINT('',(-9.86568873193234,18.6421717314713,6.1)) ;
#11257=CARTESIAN_POINT('Origin',(11.25,-19.4855715851,6.21881575202)) ;
#11258=CARTESIAN_POINT('',(9.86568873193234,-18.6421717314713,6.21881575202)) ;
#11259=CARTESIAN_POINT('Origin',(11.25,-19.4855715851,6.21881575202)) ;
#11260=CARTESIAN_POINT('',(9.54202804680158,-18.4449795386737,5.99999999999914)) ;
#11261=CARTESIAN_POINT('',(9.86568873193234,-18.6421717314713,6.21881575202)) ;
#11262=CARTESIAN_POINT('Origin',(11.25,-19.4855715851,6.)) ;
#11263=CARTESIAN_POINT('Origin',(11.25,-19.4855715851,6.1)) ;
#11264=CARTESIAN_POINT('',(9.86568873193234,-18.6421717314713,6.1)) ;
#11265=CARTESIAN_POINT('Origin',(-22.5,-7.23655192354E-15,6.21881575202)) ;
#11266=CARTESIAN_POINT('',(-21.0774386671757,0.777148798077407,6.21881575202)) ;
#11267=CARTESIAN_POINT('Origin',(-22.5,-7.23655192354E-15,6.21881575202)) ;
#11268=CARTESIAN_POINT('',(-20.7448348762197,0.958851077208162,5.99999999999914)) ;
#11269=CARTESIAN_POINT('',(-21.0774386671757,0.777148798077408,6.21881575202)) ;
#11270=CARTESIAN_POINT('Origin',(-22.5,-7.23655192354E-15,6.)) ;
#11271=CARTESIAN_POINT('Origin',(-22.5,-7.23655192354E-15,6.1)) ;
#11272=CARTESIAN_POINT('',(-21.0774386671757,0.777148798077408,6.1)) ;
#11273=CARTESIAN_POINT('Origin',(11.25,19.4855715851,6.21881575202)) ;
#11274=CARTESIAN_POINT('',(11.2117499352434,17.865022933394,6.21881575202)) ;
#11275=CARTESIAN_POINT('Origin',(11.25,19.4855715851,6.21881575202)) ;
#11276=CARTESIAN_POINT('',(11.2028068294182,17.4861284614657,5.99999999999914)) ;
#11277=CARTESIAN_POINT('',(11.2117499352434,17.865022933394,6.21881575202)) ;
#11278=CARTESIAN_POINT('Origin',(11.25,19.4855715851,6.)) ;
#11279=CARTESIAN_POINT('Origin',(11.25,19.4855715851,6.1)) ;
#11280=CARTESIAN_POINT('',(11.2117499352434,17.865022933394,6.1)) ;
#11281=CARTESIAN_POINT('Origin',(21.6506350946,-12.5,6.1)) ;
#11282=CARTESIAN_POINT('',(23.3006350946,-9.64211616751,6.2)) ;
#11283=CARTESIAN_POINT('',(20.0006350946,-15.3578838325,6.2)) ;
#11284=CARTESIAN_POINT('Origin',(21.6506350946,-12.5,6.2)) ;
#11285=CARTESIAN_POINT('',(23.3006350946,-9.64211616751,8.8)) ;
#11286=CARTESIAN_POINT('',(23.3006350946,-9.64211616751,4.24499999998)) ;
#11287=CARTESIAN_POINT('',(20.0006350946,-15.3578838325,8.8)) ;
#11288=CARTESIAN_POINT('Origin',(21.6506350946,-12.5,8.8)) ;
#11289=CARTESIAN_POINT('',(20.0006350946,-15.3578838325,4.24499999998)) ;
#11290=CARTESIAN_POINT('Origin',(21.6506350945999,-12.5000000000006,8.5000000000011)) ;
#11291=CARTESIAN_POINT('',(23.400635093838,-9.46891108630306,5.99999999999834)) ;
#11292=CARTESIAN_POINT('',(23.3506350946,-9.55551362713,6.1)) ;
#11293=CARTESIAN_POINT('',(19.9006350939093,-15.531088912845,6.00000000000624)) ;
#11294=CARTESIAN_POINT('',(19.9506350946,-15.4444863729,6.1)) ;
#11295=CARTESIAN_POINT('Origin',(21.6506350946,-12.5,6.)) ;
#11296=CARTESIAN_POINT('Origin',(-21.6506350946,-12.5,6.1)) ;
#11297=CARTESIAN_POINT('',(-20.0006350946,-15.3578838325,6.2)) ;
#11298=CARTESIAN_POINT('',(-23.3006350946,-9.64211616751,6.2)) ;
#11299=CARTESIAN_POINT('Origin',(-21.6506350946,-12.5,6.2)) ;
#11300=CARTESIAN_POINT('',(-20.0006350946,-15.3578838325,8.8)) ;
#11301=CARTESIAN_POINT('',(-20.0006350946,-15.3578838325,4.24499999998)) ;
#11302=CARTESIAN_POINT('',(-23.3006350946,-9.64211616751,8.8)) ;
#11303=CARTESIAN_POINT('Origin',(-21.6506350946,-12.5,8.8)) ;
#11304=CARTESIAN_POINT('',(-23.3006350946,-9.64211616751,4.24499999998)) ;
#11305=CARTESIAN_POINT('Origin',(-21.6506350946005,-12.4999999999996,8.5000000000011)) ;
#11306=CARTESIAN_POINT('',(-19.9006350938493,-15.5310889128105,6.00000000000579)) ;
#11307=CARTESIAN_POINT('',(-19.9506350946,-15.4444863729,6.1)) ;
#11308=CARTESIAN_POINT('',(-23.400635093898,-9.46891108633782,5.99999999999877)) ;
#11309=CARTESIAN_POINT('',(-23.3506350946,-9.55551362713,6.1)) ;
#11310=CARTESIAN_POINT('Origin',(-21.6506350946,-12.5,6.)) ;
#11311=CARTESIAN_POINT('Origin',(0.,25.,6.1)) ;
#11312=CARTESIAN_POINT('',(-3.3,25.,6.2)) ;
#11313=CARTESIAN_POINT('',(3.3,25.,6.2)) ;
#11314=CARTESIAN_POINT('Origin',(0.,25.,6.2)) ;
#11315=CARTESIAN_POINT('',(-3.3,25.,8.8)) ;
#11316=CARTESIAN_POINT('',(-3.3,25.,4.24499999998)) ;
#11317=CARTESIAN_POINT('',(3.3,25.,8.8)) ;
#11318=CARTESIAN_POINT('Origin',(0.,25.,8.8)) ;
#11319=CARTESIAN_POINT('',(3.3,25.,4.24499999998)) ;
#11320=CARTESIAN_POINT('Origin',(0.,19.4,6.)) ;
#11321=CARTESIAN_POINT('',(-3.5,27.7803887662,6.)) ;
#11322=CARTESIAN_POINT('',(-3.49999999999999,24.999999999116,6.00000000000003)) ;
#11323=CARTESIAN_POINT('',(-3.5,26.3901943831,6.)) ;
#11324=CARTESIAN_POINT('',(3.50000000000006,24.9999999991854,6.00000000000002)) ;
#11325=CARTESIAN_POINT('Origin',(8.55149284718E-14,25.,6.)) ;
#11326=CARTESIAN_POINT('',(3.5,27.7803887662,6.)) ;
#11327=CARTESIAN_POINT('',(3.5,26.3901943831,6.)) ;
#11328=CARTESIAN_POINT('',(25.8085223985,-10.8591054698,6.)) ;
#11329=CARTESIAN_POINT('Origin',(0.,0.,6.)) ;
#11330=CARTESIAN_POINT('',(24.6045787466,-10.1640082783,6.)) ;
#11331=CARTESIAN_POINT('',(22.3085223985,-16.9212832963,6.)) ;
#11332=CARTESIAN_POINT('',(21.1045787466,-16.2261861048,6.)) ;
#11333=CARTESIAN_POINT('',(-22.3085223985,-16.9212832963,6.)) ;
#11334=CARTESIAN_POINT('Origin',(0.,0.,6.)) ;
#11335=CARTESIAN_POINT('',(-21.1045787466,-16.2261861048,6.)) ;
#11336=CARTESIAN_POINT('',(-25.8085223985,-10.8591054698,6.)) ;
#11337=CARTESIAN_POINT('',(-24.6045787466,-10.1640082783,6.)) ;
#11338=CARTESIAN_POINT('Origin',(0.,0.,6.)) ;
#11339=CARTESIAN_POINT('Origin',(-1.19482201910557E-12,25.0000000000002,
8.5000000000011)) ;
#11340=CARTESIAN_POINT('',(-3.4,25.,6.1)) ;
#11341=CARTESIAN_POINT('',(3.4,25.,6.1)) ;
#11342=CARTESIAN_POINT('Origin',(26.3317240079,-11.3921161675,8.8)) ;
#11343=CARTESIAN_POINT('',(25.6743626346,-11.0125884017,8.8)) ;
#11344=CARTESIAN_POINT('',(24.4874988646,-10.3273522846,8.8)) ;
#11345=CARTESIAN_POINT('',(25.6743626346,-11.0125884017,6.2)) ;
#11346=CARTESIAN_POINT('',(24.4874988646,-10.3273522846,6.2)) ;
#11347=CARTESIAN_POINT('',(25.6743626346,-11.0125884017,7.5)) ;
#11348=CARTESIAN_POINT('Origin',(39.1,-18.7638837487,6.2)) ;
#11349=CARTESIAN_POINT('',(26.0145987277224,-11.0713657435807,6.08078462402894)) ;
#11350=CARTESIAN_POINT('Ctrl Pts',(25.8085223985027,-10.8591054698803,6.)) ;
#11351=CARTESIAN_POINT('Ctrl Pts',(25.8571374619109,-10.8871733898202,5.99999999999531)) ;
#11352=CARTESIAN_POINT('Ctrl Pts',(25.9078451689224,-10.9299496903379,6.01169150941781)) ;
#11353=CARTESIAN_POINT('Ctrl Pts',(25.9697311988347,-11.0002513821677,6.04163154551536)) ;
#11354=CARTESIAN_POINT('Ctrl Pts',(25.9947485466696,-11.0357177315965,6.05983763118273)) ;
#11355=CARTESIAN_POINT('Ctrl Pts',(26.0145987284392,-11.071365743222,6.08078462396007)) ;
#11356=CARTESIAN_POINT('Origin',(25.9243626346,-10.5795756998,5.69999999994799)) ;
#11357=CARTESIAN_POINT('Origin',(25.9243626346,-10.5795756998,13.65)) ;
#11358=CARTESIAN_POINT('',(26.3872976817,-10.7684966945,8.8)) ;
#11359=CARTESIAN_POINT('Origin',(25.9243626346,-10.5795756998,8.8)) ;
#11360=CARTESIAN_POINT('',(26.3872976817,-10.7684966945,6.5)) ;
#11361=CARTESIAN_POINT('Ctrl Pts',(26.3872976816725,-10.7684966944695,6.49999999998201)) ;
#11362=CARTESIAN_POINT('Ctrl Pts',(26.3868959264705,-10.7694811618849,6.49894607942579)) ;
#11363=CARTESIAN_POINT('Ctrl Pts',(26.3864910294718,-10.7704643512718,6.49789214772154)) ;
#11364=CARTESIAN_POINT('Ctrl Pts',(26.3659917886762,-10.8197940534219,6.44494449785955)) ;
#11365=CARTESIAN_POINT('Ctrl Pts',(26.3381799976662,-10.8652910069303,6.39277384156272)) ;
#11366=CARTESIAN_POINT('Ctrl Pts',(26.2697790282567,-10.9446832227358,6.29416151717575)) ;
#11367=CARTESIAN_POINT('Ctrl Pts',(26.2294307072862,-10.9794912243597,6.24697685916072)) ;
#11368=CARTESIAN_POINT('Ctrl Pts',(26.1340323179397,-11.037009896502,6.1579646695321)) ;
#11369=CARTESIAN_POINT('Ctrl Pts',(26.0778577824432,-11.0596414531037,6.11577330428268)) ;
#11370=CARTESIAN_POINT('Ctrl Pts',(26.0151903744484,-11.0712569093201,6.08111111750928)) ;
#11371=CARTESIAN_POINT('Ctrl Pts',(26.0148946170451,-11.0713114526719,6.0809477813369)) ;
#11372=CARTESIAN_POINT('Ctrl Pts',(26.0145987279009,-11.0713657438897,6.08078462380808)) ;
#11373=CARTESIAN_POINT('',(26.3872976817,-10.7684966945,13.65)) ;
#11374=CARTESIAN_POINT('Origin',(1.6,25.,8.8)) ;
#11375=CARTESIAN_POINT('',(22.3743626346,-16.7283560667,8.8)) ;
#11376=CARTESIAN_POINT('',(21.1874988646,-16.0431199496,8.8)) ;
#11377=CARTESIAN_POINT('',(22.5194405388,-17.4678217823,8.8)) ;
#11378=CARTESIAN_POINT('Origin',(0.,0.,8.8)) ;
#11379=CARTESIAN_POINT('Origin',(22.1243626346,-17.1613687686,8.8)) ;
#11380=CARTESIAN_POINT('Origin',(0.,0.,6.5)) ;
#11381=CARTESIAN_POINT('',(-22.5194405388,-17.4678217823,6.5)) ;
#11382=CARTESIAN_POINT('',(13.6636278502198,-25.0111030138756,6.5)) ;
#11383=CARTESIAN_POINT('Origin',(0.,0.,6.5)) ;
#11384=CARTESIAN_POINT('',(-22.5953833524105,-16.9936204957114,6.08078462405313)) ;
#11385=CARTESIAN_POINT('Ctrl Pts',(-22.5194405388094,-17.4678217823238,
6.49999999998684)) ;
#11386=CARTESIAN_POINT('Ctrl Pts',(-22.5200922359486,-17.4669816171815,
6.4989460778956)) ;
#11387=CARTESIAN_POINT('Ctrl Pts',(-22.5207412548291,-17.4661393709141,
6.49789214978989)) ;
#11388=CARTESIAN_POINT('Ctrl Pts',(-22.553212395341,-17.4237216746888,6.44494446983119)) ;
#11389=CARTESIAN_POINT('Ctrl Pts',(-22.5787080290974,-17.3768874659649,
6.39277384396564)) ;
#11390=CARTESIAN_POINT('Ctrl Pts',(-22.613263219733,-17.2779543852514,6.29416152319963)) ;
#11391=CARTESIAN_POINT('Ctrl Pts',(-22.6232336733237,-17.2256077153181,
6.24697686637815)) ;
#11392=CARTESIAN_POINT('Ctrl Pts',(-22.625347112133,-17.1142309518581,6.1579646764134)) ;
#11393=CARTESIAN_POINT('Ctrl Pts',(-22.6168593483308,-17.0542665979326,
6.1157733099033)) ;
#11394=CARTESIAN_POINT('Ctrl Pts',(-22.5955849243286,-16.9941872989761,
6.08111112043804)) ;
#11395=CARTESIAN_POINT('Ctrl Pts',(-22.595484280663,-16.9939038913557,6.08094778281178)) ;
#11396=CARTESIAN_POINT('Ctrl Pts',(-22.5953833527674,-16.9936204957115,
6.08078462383227)) ;
#11397=CARTESIAN_POINT('Ctrl Pts',(-22.3085223985144,-16.9212832963396,
6.)) ;
#11398=CARTESIAN_POINT('Ctrl Pts',(-22.3571374619185,-16.9493512162867,
5.99999999999643)) ;
#11399=CARTESIAN_POINT('Ctrl Pts',(-22.4195366783519,-16.9718772284684,
6.01169150941781)) ;
#11400=CARTESIAN_POINT('Ctrl Pts',(-22.511362744377,-16.9903212565999,6.0416315455203)) ;
#11401=CARTESIAN_POINT('Ctrl Pts',(-22.5545861778974,-16.9942537406455,
6.05983763119696)) ;
#11402=CARTESIAN_POINT('Ctrl Pts',(-22.5953833524583,-16.9936204965115,
6.08078462398426)) ;
#11403=CARTESIAN_POINT('',(22.5953833523902,-16.9936204956541,6.08078462402019)) ;
#11404=CARTESIAN_POINT('Ctrl Pts',(22.3085223985585,-16.9212832962815,6.)) ;
#11405=CARTESIAN_POINT('Ctrl Pts',(22.357137461962,-16.9493512162294,5.99999999999543)) ;
#11406=CARTESIAN_POINT('Ctrl Pts',(22.4195366783959,-16.9718772284103,6.01169150941781)) ;
#11407=CARTESIAN_POINT('Ctrl Pts',(22.5113627444003,-16.9903212565376,6.04163154551358)) ;
#11408=CARTESIAN_POINT('Ctrl Pts',(22.5545861778961,-16.9942537405836,6.05983763117759)) ;
#11409=CARTESIAN_POINT('Ctrl Pts',(22.595383352438,-16.9936204964542,6.08078462395134)) ;
#11410=CARTESIAN_POINT('',(22.5194405388,-17.4678217823,6.5)) ;
#11411=CARTESIAN_POINT('Ctrl Pts',(22.5194405388094,-17.4678217823238,6.49999999998684)) ;
#11412=CARTESIAN_POINT('Ctrl Pts',(22.5200922359489,-17.466981617181,6.49894607789501)) ;
#11413=CARTESIAN_POINT('Ctrl Pts',(22.5207412548294,-17.4661393709138,6.49789214979062)) ;
#11414=CARTESIAN_POINT('Ctrl Pts',(22.5532123953377,-17.423721674693,6.444944469824)) ;
#11415=CARTESIAN_POINT('Ctrl Pts',(22.5787080290974,-17.3768874659648,6.3927738439656)) ;
#11416=CARTESIAN_POINT('Ctrl Pts',(22.6132632197329,-17.2779543852517,6.29416152319988)) ;
#11417=CARTESIAN_POINT('Ctrl Pts',(22.6232336733236,-17.2256077153185,6.24697686637843)) ;
#11418=CARTESIAN_POINT('Ctrl Pts',(22.625347112133,-17.1142309518585,6.15796467641363)) ;
#11419=CARTESIAN_POINT('Ctrl Pts',(22.6168593483308,-17.0542665979329,6.11577330990351)) ;
#11420=CARTESIAN_POINT('Ctrl Pts',(22.5955849243219,-16.9941872989572,6.08111112042713)) ;
#11421=CARTESIAN_POINT('Ctrl Pts',(22.5954842806494,-16.9939038913176,6.08094778278984)) ;
#11422=CARTESIAN_POINT('Ctrl Pts',(22.595383352747,-16.9936204956542,6.0807846237993)) ;
#11423=CARTESIAN_POINT('Origin',(0.,0.,6.5)) ;
#11424=CARTESIAN_POINT('Origin',(20.0006350946,-15.3578838325,8.8)) ;
#11425=CARTESIAN_POINT('',(22.3743626346,-16.7283560667,6.2)) ;
#11426=CARTESIAN_POINT('',(21.1874988646,-16.0431199496,6.2)) ;
#11427=CARTESIAN_POINT('',(22.3743626346,-16.7283560667,7.5)) ;
#11428=CARTESIAN_POINT('Origin',(-39.1,18.7638837487,6.2)) ;
#11429=CARTESIAN_POINT('Origin',(22.1243626346,-17.1613687686,5.69999999991353)) ;
#11430=CARTESIAN_POINT('Origin',(22.1243626346,-17.1613687686,13.65)) ;
#11431=CARTESIAN_POINT('',(22.5194405388,-17.4678217823,13.65)) ;
#11432=CARTESIAN_POINT('Origin',(-23.0317240079,-17.1078838325,8.8)) ;
#11433=CARTESIAN_POINT('',(-22.3743626346,-16.7283560667,8.8)) ;
#11434=CARTESIAN_POINT('',(-21.1874988646,-16.0431199496,8.8)) ;
#11435=CARTESIAN_POINT('',(-22.3743626346,-16.7283560667,6.2)) ;
#11436=CARTESIAN_POINT('',(-21.1874988646,-16.0431199496,6.2)) ;
#11437=CARTESIAN_POINT('',(-22.3743626346,-16.7283560667,7.5)) ;
#11438=CARTESIAN_POINT('Origin',(-39.3,-26.5003773558,6.2)) ;
#11439=CARTESIAN_POINT('Origin',(-22.1243626346,-17.1613687686,5.69999999998591)) ;
#11440=CARTESIAN_POINT('Origin',(-22.1243626346,-17.1613687686,13.65)) ;
#11441=CARTESIAN_POINT('',(-22.5194405388,-17.4678217823,8.8)) ;
#11442=CARTESIAN_POINT('Origin',(-22.1243626346,-17.1613687686,8.8)) ;
#11443=CARTESIAN_POINT('',(-22.5194405388,-17.4678217823,13.65)) ;
#11444=CARTESIAN_POINT('Origin',(1.6,25.,8.8)) ;
#11445=CARTESIAN_POINT('',(-25.6743626346,-11.0125884017,8.8)) ;
#11446=CARTESIAN_POINT('',(-24.4874988646,-10.3273522846,8.8)) ;
#11447=CARTESIAN_POINT('',(-26.3872976817,-10.7684966945,8.8)) ;
#11448=CARTESIAN_POINT('Origin',(0.,0.,8.8)) ;
#11449=CARTESIAN_POINT('Origin',(-25.9243626346,-10.5795756998,8.8)) ;
#11450=CARTESIAN_POINT('Origin',(0.,0.,6.5)) ;
#11451=CARTESIAN_POINT('',(-3.86785714286,28.2363184768,6.5)) ;
#11452=CARTESIAN_POINT('',(-26.3872976817,-10.7684966945,6.5)) ;
#11453=CARTESIAN_POINT('Origin',(0.,0.,6.5)) ;
#11454=CARTESIAN_POINT('',(-3.41921537541075,28.0649862395495,6.08078462418545)) ;
#11455=CARTESIAN_POINT('Ctrl Pts',(-3.86785714285896,28.2363184767851,6.49999999999899)) ;
#11456=CARTESIAN_POINT('Ctrl Pts',(-3.86680369034399,28.2364627804357,6.49894607831917)) ;
#11457=CARTESIAN_POINT('Ctrl Pts',(-3.8657497744286,28.2366037241107,6.49789214922878)) ;
#11458=CARTESIAN_POINT('Ctrl Pts',(-3.81277939497464,28.2435157095405,6.44494447730782)) ;
#11459=CARTESIAN_POINT('Ctrl Pts',(-3.75947196890609,28.2421784708253,6.39277384320122)) ;
#11460=CARTESIAN_POINT('Ctrl Pts',(-3.65651581132869,28.2226376028753,6.29416152144487)) ;
#11461=CARTESIAN_POINT('Ctrl Pts',(-3.6061970381645,28.205098933633,6.24697686427605)) ;
#11462=CARTESIAN_POINT('Ctrl Pts',(-3.50868521221608,28.1512408428583,6.1579646744094)) ;
#11463=CARTESIAN_POINT('Ctrl Pts',(-3.46099844065362,28.1139080466909,6.11577330826644)) ;
#11464=CARTESIAN_POINT('Ctrl Pts',(-3.41960545444015,28.0654442061972,6.08111111963159)) ;
#11465=CARTESIAN_POINT('Ctrl Pts',(-3.41941033863507,28.0652153430729,6.08094778247512)) ;
#11466=CARTESIAN_POINT('Ctrl Pts',(-3.41921537531581,28.0649862397878,6.08078462396436)) ;
#11467=CARTESIAN_POINT('Ctrl Pts',(-3.5,27.7803887661782,6.)) ;
#11468=CARTESIAN_POINT('Ctrl Pts',(-3.49999999999759,27.8365246060662,6.00000000000241)) ;
#11469=CARTESIAN_POINT('Ctrl Pts',(-3.48830849058219,27.9018269187647,6.01169150941781)) ;
#11470=CARTESIAN_POINT('Ctrl Pts',(-3.45836845445844,27.9905726388008,6.04163154554156)) ;
#11471=CARTESIAN_POINT('Ctrl Pts',(-3.44016236874182,28.0299714723576,6.05983763125818)) ;
#11472=CARTESIAN_POINT('Ctrl Pts',(-3.41921537591168,28.0649862399073,6.08078462408832)) ;
#11473=CARTESIAN_POINT('',(-26.0145987277821,-11.0713657435697,6.08078462406189)) ;
#11474=CARTESIAN_POINT('Ctrl Pts',(-25.808522398531,-10.8591054698131,6.)) ;
#11475=CARTESIAN_POINT('Ctrl Pts',(-25.8571374619387,-10.8871733897539,
5.99999999999631)) ;
#11476=CARTESIAN_POINT('Ctrl Pts',(-25.9078451689507,-10.9299496902707,
6.01169150941781)) ;
#11477=CARTESIAN_POINT('Ctrl Pts',(-25.969731198877,-11.0002513821164,6.04163154552208)) ;
#11478=CARTESIAN_POINT('Ctrl Pts',(-25.9947485467239,-11.0357177315667,
6.0598376312021)) ;
#11479=CARTESIAN_POINT('Ctrl Pts',(-26.0145987284989,-11.071365743211,6.080784623993)) ;
#11480=CARTESIAN_POINT('Ctrl Pts',(-26.3872976816725,-10.7684966944695,
6.49999999998201)) ;
#11481=CARTESIAN_POINT('Ctrl Pts',(-26.3868959264705,-10.769481161885,6.49894607942567)) ;
#11482=CARTESIAN_POINT('Ctrl Pts',(-26.3864910294717,-10.7704643512721,
6.49789214772128)) ;
#11483=CARTESIAN_POINT('Ctrl Pts',(-26.3659917886761,-10.8197940534221,
6.44494449785881)) ;
#11484=CARTESIAN_POINT('Ctrl Pts',(-26.3381799976659,-10.8652910069308,
6.39277384156219)) ;
#11485=CARTESIAN_POINT('Ctrl Pts',(-26.2697790282562,-10.9446832227363,
6.29416151717512)) ;
#11486=CARTESIAN_POINT('Ctrl Pts',(-26.2294307072856,-10.9794912243601,
6.24697685916004)) ;
#11487=CARTESIAN_POINT('Ctrl Pts',(-26.134032317939,-11.0370098965024,6.15796466953148)) ;
#11488=CARTESIAN_POINT('Ctrl Pts',(-26.0778577824424,-11.0596414531039,
6.11577330428219)) ;
#11489=CARTESIAN_POINT('Ctrl Pts',(-26.0151903744678,-11.0712569093164,
6.08111111752002)) ;
#11490=CARTESIAN_POINT('Ctrl Pts',(-26.0148946170847,-11.0713114526646,
6.08094778135875)) ;
#11491=CARTESIAN_POINT('Ctrl Pts',(-26.0145987279606,-11.0713657438788,
6.08078462384101)) ;
#11492=CARTESIAN_POINT('Origin',(-23.3006350946,-9.64211616751,8.8)) ;
#11493=CARTESIAN_POINT('',(-25.6743626346,-11.0125884017,6.2)) ;
#11494=CARTESIAN_POINT('',(-24.4874988646,-10.3273522846,6.2)) ;
#11495=CARTESIAN_POINT('',(-25.6743626346,-11.0125884017,7.5)) ;
#11496=CARTESIAN_POINT('Origin',(39.3,26.5003773558,6.2)) ;
#11497=CARTESIAN_POINT('Origin',(-25.9243626346,-10.5795756998,5.70000000002037)) ;
#11498=CARTESIAN_POINT('Origin',(0.,0.,10.5000000001)) ;
#11499=CARTESIAN_POINT('',(13.6636278502198,-25.0111030138756,10.5000000001)) ;
#11500=CARTESIAN_POINT('',(3.86785714286,28.2363184768,6.5)) ;
#11501=CARTESIAN_POINT('Origin',(0.,0.,6.5)) ;
#11502=CARTESIAN_POINT('',(3.86785714286,28.2363184768,8.8)) ;
#11503=CARTESIAN_POINT('',(3.86785714286,28.2363184768,13.65)) ;
#11504=CARTESIAN_POINT('',(-3.86785714286,28.2363184768,8.8)) ;
#11505=CARTESIAN_POINT('Origin',(0.,0.,8.8)) ;
#11506=CARTESIAN_POINT('',(-3.86785714286,28.2363184768,13.65)) ;
#11507=CARTESIAN_POINT('',(-26.3872976817,-10.7684966945,13.65)) ;
#11508=CARTESIAN_POINT('Origin',(-25.9243626346,-10.5795756998,13.65)) ;
#11509=CARTESIAN_POINT('Origin',(-3.3,28.5,8.8)) ;
#11510=CARTESIAN_POINT('',(-3.3,27.7409444684,8.8)) ;
#11511=CARTESIAN_POINT('',(-3.3,26.3704722342,8.8)) ;
#11512=CARTESIAN_POINT('',(-3.3,27.7409444684,6.2)) ;
#11513=CARTESIAN_POINT('',(-3.3,26.3704722342,6.2)) ;
#11514=CARTESIAN_POINT('',(-3.3,27.7409444684,7.5)) ;
#11515=CARTESIAN_POINT('Origin',(-3.3,38.9658268293,6.2)) ;
#11516=CARTESIAN_POINT('Origin',(-3.8,27.7409444684,5.7)) ;
#11517=CARTESIAN_POINT('Origin',(-3.8,27.7409444684,13.65)) ;
#11518=CARTESIAN_POINT('Origin',(-3.8,27.7409444684,8.8)) ;
#11519=CARTESIAN_POINT('Origin',(1.6,25.,8.8)) ;
#11520=CARTESIAN_POINT('',(3.3,27.7409444684,8.8)) ;
#11521=CARTESIAN_POINT('',(3.3,26.3704722342,8.8)) ;
#11522=CARTESIAN_POINT('Origin',(3.8,27.7409444684,8.8)) ;
#11523=CARTESIAN_POINT('Origin',(3.3,25.,8.8)) ;
#11524=CARTESIAN_POINT('',(3.3,27.7409444684,6.2)) ;
#11525=CARTESIAN_POINT('',(3.3,26.3704722342,6.2)) ;
#11526=CARTESIAN_POINT('',(3.3,27.7409444684,7.5)) ;
#11527=CARTESIAN_POINT('Origin',(3.3,-39.1609711382,6.2)) ;
#11528=CARTESIAN_POINT('',(3.41921537541076,28.0649862395495,6.08078462418545)) ;
#11529=CARTESIAN_POINT('Ctrl Pts',(3.50000000000001,27.7803887661782,6.)) ;
#11530=CARTESIAN_POINT('Ctrl Pts',(3.49999999999738,27.8415860360952,6.00000000000263)) ;
#11531=CARTESIAN_POINT('Ctrl Pts',(3.48615657642937,27.9123650701724,6.01384342357064)) ;
#11532=CARTESIAN_POINT('Ctrl Pts',(3.45400358048058,27.9999583028243,6.04599641951943)) ;
#11533=CARTESIAN_POINT('Ctrl Pts',(3.43785569939262,28.0338272759916,6.06214430060739)) ;
#11534=CARTESIAN_POINT('Ctrl Pts',(3.41921537591169,28.0649862399073,6.08078462408832)) ;
#11535=CARTESIAN_POINT('Origin',(3.8,27.7409444684,5.70000000000001)) ;
#11536=CARTESIAN_POINT('Origin',(0.,0.,6.5)) ;
#11537=CARTESIAN_POINT('Ctrl Pts',(3.86785714285897,28.2363184767851,6.49999999999899)) ;
#11538=CARTESIAN_POINT('Ctrl Pts',(3.86680369034378,28.2364627804357,6.49894607831896)) ;
#11539=CARTESIAN_POINT('Ctrl Pts',(3.86574977442877,28.2366037241107,6.49789214922897)) ;
#11540=CARTESIAN_POINT('Ctrl Pts',(3.81277939497492,28.2435157095405,6.44494447730793)) ;
#11541=CARTESIAN_POINT('Ctrl Pts',(3.75947196890666,28.2421784708253,6.39277384320178)) ;
#11542=CARTESIAN_POINT('Ctrl Pts',(3.65651581132985,28.2226376028756,6.29416152144597)) ;
#11543=CARTESIAN_POINT('Ctrl Pts',(3.60619703816588,28.2050989336335,6.24697686427737)) ;
#11544=CARTESIAN_POINT('Ctrl Pts',(3.50868521221741,28.1512408428593,6.15796467441062)) ;
#11545=CARTESIAN_POINT('Ctrl Pts',(3.46099844065479,28.113908046692,6.11577330826745)) ;
#11546=CARTESIAN_POINT('Ctrl Pts',(3.41960545444078,28.065444206198,6.08111111963212)) ;
#11547=CARTESIAN_POINT('Ctrl Pts',(3.41941033863539,28.0652153430733,6.08094778247539)) ;
#11548=CARTESIAN_POINT('Ctrl Pts',(3.41921537531581,28.0649862397878,6.08078462396436)) ;
#11549=CARTESIAN_POINT('Origin',(3.8,27.7409444684,13.65)) ;
#13478=UNCERTAINTY_MEASURE_WITH_UNIT(LENGTH_MEASURE(0.01),#13511,
'DISTANCE_ACCURACY_VALUE',
'Maximum model space distance between geometric entities at asserted c
onnectivities') ;
#13493=UNCERTAINTY_MEASURE_WITH_UNIT(LENGTH_MEASURE(0.01),#13511,
'DISTANCE_ACCURACY_VALUE',
'Maximum model space distance between geometric entities at asserted c
onnectivities') ;
#13495=(
GEOMETRIC_REPRESENTATION_CONTEXT(3)
GLOBAL_UNCERTAINTY_ASSIGNED_CONTEXT((#13478))
GLOBAL_UNIT_ASSIGNED_CONTEXT((#13511,#13513,#13514))
REPRESENTATION_CONTEXT('','3D')
) ;
#13510=(
GEOMETRIC_REPRESENTATION_CONTEXT(3)
GLOBAL_UNCERTAINTY_ASSIGNED_CONTEXT((#13493))
GLOBAL_UNIT_ASSIGNED_CONTEXT((#13511,#13513,#13514))
REPRESENTATION_CONTEXT('','3D')
) ;
#13511=(
LENGTH_UNIT()
NAMED_UNIT(*)
SI_UNIT(.MILLI.,.METRE.)
) ;
#13513=(
NAMED_UNIT(*)
PLANE_ANGLE_UNIT()
SI_UNIT($,.RADIAN.)
) ;
#13514=(
NAMED_UNIT(*)
SI_UNIT($,.STERADIAN.)
SOLID_ANGLE_UNIT()
) ;
#13516=SHAPE_DEFINITION_REPRESENTATION(#13532,#13563) ;
#13532=PRODUCT_DEFINITION_SHAPE('',$,#13580) ;
#13563=SHAPE_REPRESENTATION('',(#7571),#13495) ;
#13578=PRODUCT_DEFINITION_CONTEXT('part definition',#13628,'design') ;
#13580=PRODUCT_DEFINITION('Front_End_Cap','Front_End_Cap',#13596,#13578) ;
#13596=PRODUCT_DEFINITION_FORMATION('',$,#13631) ;
#13628=APPLICATION_CONTEXT(
'Core Data for Automotive Mechanical Design Process') ;
#13629=PRODUCT_CONTEXT('part definition',#13628,'mechanical') ;
#13631=PRODUCT('Front_End_Cap','Front_End_Cap',$,(#13629)) ;
#13647=PRESENTATION_STYLE_ASSIGNMENT((#13652)) ;
#13652=SURFACE_STYLE_USAGE(.BOTH.,#13657) ;
#13657=SURFACE_SIDE_STYLE('',(#13662)) ;
#13662=SURFACE_STYLE_FILL_AREA(#13667) ;
#13667=FILL_AREA_STYLE('Opaque(245,245,246)',(#13672)) ;
#13672=FILL_AREA_STYLE_COLOUR('Opaque(245,245,246)',#13677) ;
#13677=COLOUR_RGB('Opaque(245,245,246)', 0.09019608, 0.27058824, 0.51372549) ;
ENDSEC;
END-ISO-10303-21;
